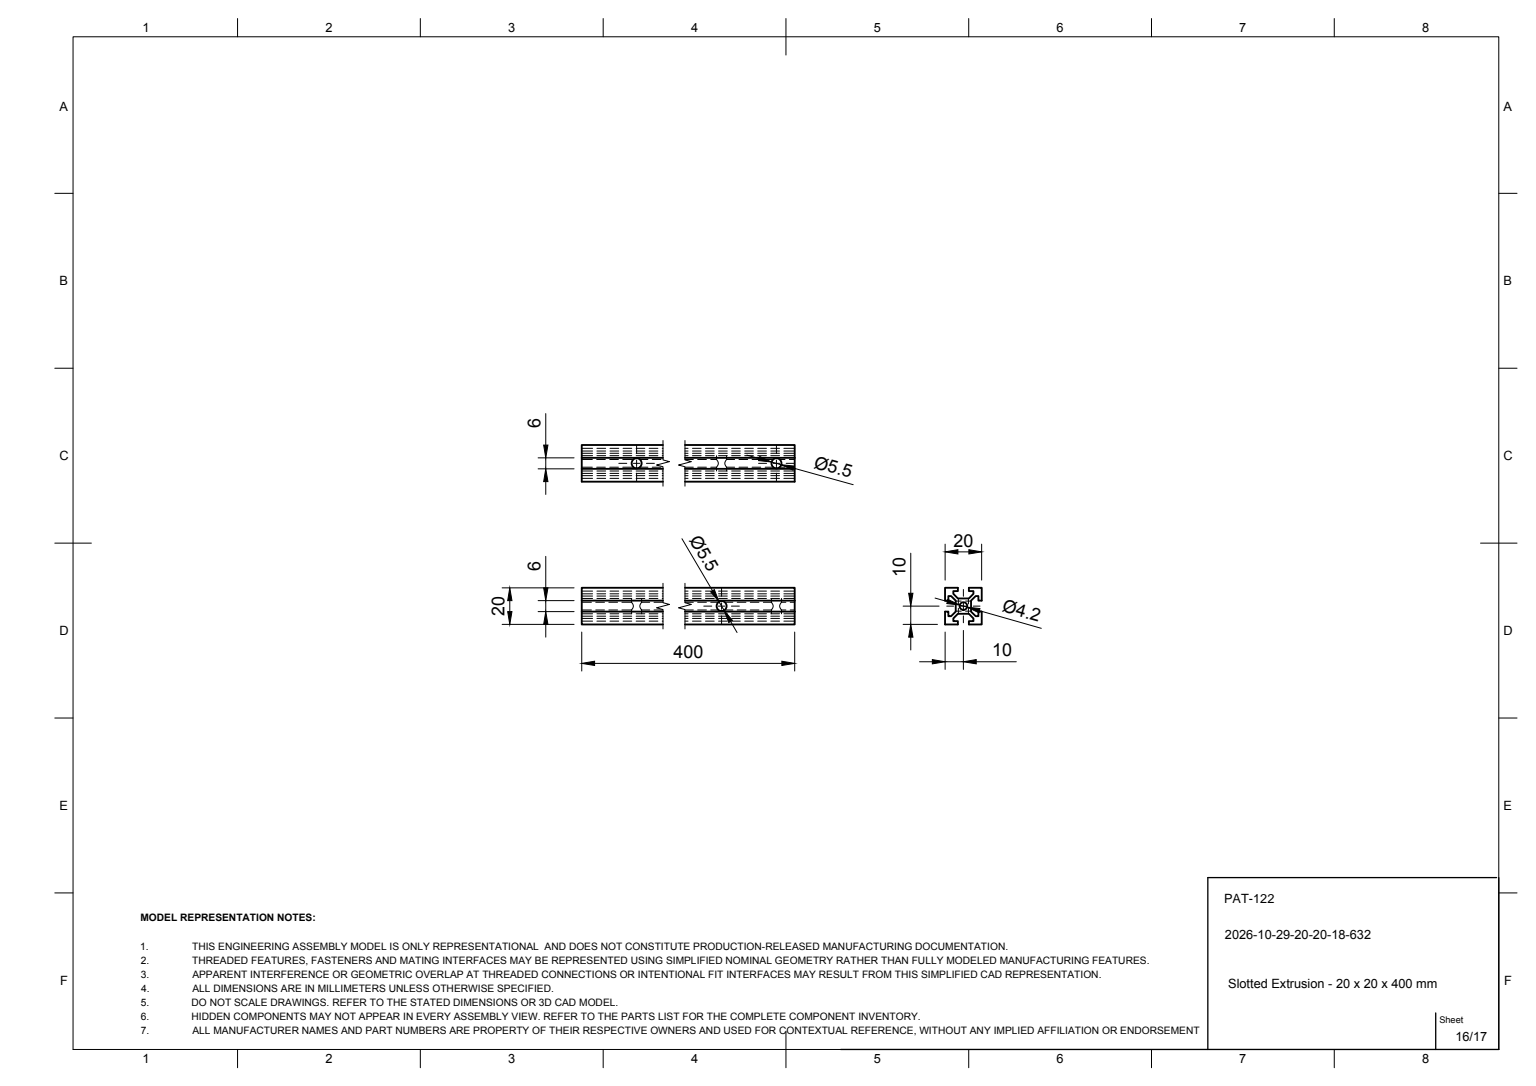
ISO-10303-21;
HEADER;
/* Generated by software containing ST-Developer
 * from STEP Tools, Inc. (www.steptools.com) 
 */

FILE_DESCRIPTION(
/* description */ ('PAT-122'),
/* implementation_level */ '2;1');

FILE_NAME(
/* name */ 'Slotted Extrusion - 20 x 20 x 400 mm.step',
/* time_stamp */ '2026-10-29T20:20:12-07:00',
/* author */ (''),
/* organization */ (''),
/* preprocessor_version */ 'ST-DEVELOPER v20.2',
/* originating_system */ 'Autodesk Translation Framework v15.17.0.0',
/* authorisation */ '');

FILE_SCHEMA (('AUTOMOTIVE_DESIGN { 1 0 10303 214 3 1 1 }'));
ENDSEC;

DATA;
#10=MECHANICAL_DESIGN_GEOMETRIC_PRESENTATION_REPRESENTATION('',(#504),#10019);
#425=B_SPLINE_CURVE_WITH_KNOTS('',3,(#8517,#8518,#8519,#8520,#8521,#8522,
#8523,#8524,#8525,#8526,#8527,#8528),.UNSPECIFIED.,.F.,.F.,(4,2,2,2,2,4),
(0.671876099962389,0.714365153473771,0.756854206985153,0.841832314007917,
0.92482323197575,1.00781414994358),.UNSPECIFIED.);
#426=B_SPLINE_CURVE_WITH_KNOTS('',3,(#8530,#8531,#8532,#8533,#8534,#8535,
#8536,#8537,#8538,#8539,#8540,#8541),.UNSPECIFIED.,.F.,.F.,(4,2,2,2,2,4),
(0.335938049981194,0.418928967949028,0.501919885916861,0.586897992939625,
0.629387046451007,0.671876099962389),.UNSPECIFIED.);
#427=B_SPLINE_CURVE_WITH_KNOTS('',3,(#8546,#8547,#8548,#8549,#8550,#8551,
#8552,#8553,#8554,#8555,#8556,#8557),.UNSPECIFIED.,.F.,.F.,(4,2,2,2,2,4),
(0.,0.042489053511382,0.0849781070227641,0.169956214045528,0.252947132013361,
0.335938049981194),.UNSPECIFIED.);
#428=B_SPLINE_CURVE_WITH_KNOTS('',3,(#8558,#8559,#8560,#8561,#8562,#8563,
#8564,#8565,#8566,#8567,#8568,#8569),.UNSPECIFIED.,.F.,.F.,(4,2,2,2,2,4),
(1.00781414994358,1.09080506791142,1.17379598587925,1.25877409290201,1.3012631464134,
1.34375219992478),.UNSPECIFIED.);
#429=B_SPLINE_CURVE_WITH_KNOTS('',3,(#8572,#8573,#8574,#8575,#8576,#8577,
#8578,#8579,#8580,#8581,#8582,#8583,#8584,#8585,#8586,#8587,#8588,#8589,
#8590,#8591,#8592,#8593),.UNSPECIFIED.,.F.,.F.,(4,2,2,2,2,2,2,2,2,2,4),
(0.,0.0424890535113821,0.0849781070227642,0.169956214045528,0.252947132013361,
0.335938049981194,0.418928967949028,0.501919885916861,0.586897992939625,
0.629387046451007,0.671876099962389),.UNSPECIFIED.);
#430=B_SPLINE_CURVE_WITH_KNOTS('',3,(#8594,#8595,#8596,#8597,#8598,#8599,
#8600,#8601,#8602,#8603,#8604,#8605,#8606,#8607,#8608,#8609,#8610,#8611,
#8612,#8613,#8614,#8615),.UNSPECIFIED.,.F.,.F.,(4,2,2,2,2,2,2,2,2,2,4),
(0.671876099962389,0.714365153473771,0.756854206985153,0.841832314007917,
0.92482323197575,1.00781414994358,1.09080506791142,1.17379598587925,1.25877409290201,
1.3012631464134,1.34375219992478),.UNSPECIFIED.);
#431=B_SPLINE_CURVE_WITH_KNOTS('',3,(#8622,#8623,#8624,#8625,#8626,#8627,
#8628,#8629,#8630,#8631,#8632,#8633),.UNSPECIFIED.,.F.,.F.,(4,2,2,2,2,4),
(0.67187609996239,0.714365153473772,0.756854206985154,0.841832314007918,
0.924823231975752,1.00781414994359),.UNSPECIFIED.);
#432=B_SPLINE_CURVE_WITH_KNOTS('',3,(#8635,#8636,#8637,#8638,#8639,#8640,
#8641,#8642,#8643,#8644,#8645,#8646),.UNSPECIFIED.,.F.,.F.,(4,2,2,2,2,4),
(0.335938049981195,0.418928967949029,0.501919885916863,0.586897992939627,
0.629387046451009,0.67187609996239),.UNSPECIFIED.);
#433=B_SPLINE_CURVE_WITH_KNOTS('',3,(#8651,#8652,#8653,#8654,#8655,#8656,
#8657,#8658,#8659,#8660,#8661,#8662),.UNSPECIFIED.,.F.,.F.,(4,2,2,2,2,4),
(0.,0.042489053511382,0.0849781070227639,0.169956214045528,0.252947132013362,
0.335938049981195),.UNSPECIFIED.);
#434=B_SPLINE_CURVE_WITH_KNOTS('',3,(#8663,#8664,#8665,#8666,#8667,#8668,
#8669,#8670,#8671,#8672,#8673,#8674),.UNSPECIFIED.,.F.,.F.,(4,2,2,2,2,4),
(1.00781414994359,1.09080506791142,1.17379598587925,1.25877409290202,1.3012631464134,
1.34375219992478),.UNSPECIFIED.);
#435=B_SPLINE_CURVE_WITH_KNOTS('',3,(#8677,#8678,#8679,#8680,#8681,#8682,
#8683,#8684,#8685,#8686,#8687,#8688,#8689,#8690,#8691,#8692,#8693,#8694,
#8695,#8696,#8697,#8698),.UNSPECIFIED.,.F.,.F.,(4,2,2,2,2,2,2,2,2,2,4),
(0.,0.042489053511382,0.084978107022764,0.169956214045528,0.252947132013362,
0.335938049981195,0.418928967949029,0.501919885916863,0.586897992939627,
0.629387046451009,0.671876099962391),.UNSPECIFIED.);
#436=B_SPLINE_CURVE_WITH_KNOTS('',3,(#8699,#8700,#8701,#8702,#8703,#8704,
#8705,#8706,#8707,#8708,#8709,#8710,#8711,#8712,#8713,#8714,#8715,#8716,
#8717,#8718,#8719,#8720),.UNSPECIFIED.,.F.,.F.,(4,2,2,2,2,2,2,2,2,2,4),
(0.671876099962391,0.714365153473772,0.756854206985154,0.841832314007918,
0.924823231975752,1.00781414994359,1.09080506791142,1.17379598587925,1.25877409290202,
1.3012631464134,1.34375219992478),.UNSPECIFIED.);
#437=B_SPLINE_CURVE_WITH_KNOTS('',3,(#8726,#8727,#8728,#8729,#8730,#8731,
#8732,#8733,#8734,#8735,#8736,#8737,#8738,#8739,#8740,#8741,#8742,#8743,
#8744,#8745,#8746,#8747,#8748,#8749,#8750,#8751,#8752,#8753,#8754,#8755,
#8756,#8757),.UNSPECIFIED.,.F.,.F.,(4,2,2,2,2,2,2,2,2,2,2,2,2,2,2,4),(0.,
0.0424890535113821,0.0849781070227642,0.169956214045528,0.252947132013362,
0.335938049981195,0.418928967949028,0.501919885916861,0.586897992939625,
0.629387046451007,0.67187609996239,0.714365153473772,0.756854206985154,
0.841832314007918,0.924823231975751,1.00781414994358),.UNSPECIFIED.);
#438=B_SPLINE_CURVE_WITH_KNOTS('',3,(#8759,#8760,#8761,#8762,#8763,#8764,
#8765,#8766,#8767,#8768,#8769,#8770),.UNSPECIFIED.,.F.,.F.,(4,2,2,2,2,4),
(1.00781414994358,1.09080506791142,1.17379598587925,1.25877409290201,1.3012631464134,
1.34375219992478),.UNSPECIFIED.);
#439=B_SPLINE_CURVE_WITH_KNOTS('',3,(#8777,#8778,#8779,#8780,#8781,#8782,
#8783,#8784,#8785,#8786,#8787,#8788,#8789,#8790,#8791,#8792,#8793,#8794,
#8795,#8796,#8797,#8798),.UNSPECIFIED.,.F.,.F.,(4,2,2,2,2,2,2,2,2,2,4),
(0.335938049981195,0.418928967949028,0.501919885916861,0.586897992939625,
0.629387046451007,0.671876099962389,0.714365153473771,0.756854206985153,
0.841832314007918,0.924823231975751,1.00781414994358),.UNSPECIFIED.);
#440=B_SPLINE_CURVE_WITH_KNOTS('',3,(#8803,#8804,#8805,#8806,#8807,#8808,
#8809,#8810,#8811,#8812,#8813,#8814),.UNSPECIFIED.,.F.,.F.,(4,2,2,2,2,4),
(0.,0.0424890535113821,0.0849781070227642,0.169956214045528,0.252947132013361,
0.335938049981195),.UNSPECIFIED.);
#441=B_SPLINE_CURVE_WITH_KNOTS('',3,(#8815,#8816,#8817,#8818,#8819,#8820,
#8821,#8822,#8823,#8824,#8825,#8826),.UNSPECIFIED.,.F.,.F.,(4,2,2,2,2,4),
(1.00781414994358,1.09080506791142,1.17379598587925,1.25877409290201,1.3012631464134,
1.34375219992478),.UNSPECIFIED.);
#442=B_SPLINE_CURVE_WITH_KNOTS('',3,(#8833,#8834,#8835,#8836,#8837,#8838,
#8839,#8840,#8841,#8842,#8843,#8844,#8845,#8846,#8847,#8848,#8849,#8850,
#8851,#8852,#8853,#8854),.UNSPECIFIED.,.F.,.F.,(4,2,2,2,2,2,2,2,2,2,4),
(0.335938049981195,0.418928967949029,0.501919885916863,0.586897992939627,
0.629387046451009,0.67187609996239,0.714365153473772,0.756854206985154,
0.841832314007918,0.924823231975752,1.00781414994359),.UNSPECIFIED.);
#443=B_SPLINE_CURVE_WITH_KNOTS('',3,(#8859,#8860,#8861,#8862,#8863,#8864,
#8865,#8866,#8867,#8868,#8869,#8870),.UNSPECIFIED.,.F.,.F.,(4,2,2,2,2,4),
(0.,0.042489053511382,0.0849781070227639,0.169956214045528,0.252947132013361,
0.335938049981195),.UNSPECIFIED.);
#444=B_SPLINE_CURVE_WITH_KNOTS('',3,(#8871,#8872,#8873,#8874,#8875,#8876,
#8877,#8878,#8879,#8880,#8881,#8882),.UNSPECIFIED.,.F.,.F.,(4,2,2,2,2,4),
(1.00781414994359,1.09080506791142,1.17379598587925,1.25877409290202,1.3012631464134,
1.34375219992478),.UNSPECIFIED.);
#445=B_SPLINE_CURVE_WITH_KNOTS('',3,(#8885,#8886,#8887,#8888,#8889,#8890,
#8891,#8892,#8893,#8894,#8895,#8896,#8897,#8898,#8899,#8900,#8901,#8902,
#8903,#8904,#8905,#8906,#8907,#8908,#8909,#8910,#8911,#8912,#8913,#8914,
#8915,#8916),.UNSPECIFIED.,.F.,.F.,(4,2,2,2,2,2,2,2,2,2,2,2,2,2,2,4),(0.,
0.042489053511382,0.084978107022764,0.169956214045528,0.252947132013362,
0.335938049981195,0.418928967949029,0.501919885916863,0.586897992939627,
0.629387046451009,0.671876099962391,0.714365153473772,0.756854206985154,
0.841832314007918,0.924823231975752,1.00781414994359),.UNSPECIFIED.);
#446=B_SPLINE_CURVE_WITH_KNOTS('',3,(#8917,#8918,#8919,#8920,#8921,#8922,
#8923,#8924,#8925,#8926,#8927,#8928),.UNSPECIFIED.,.F.,.F.,(4,2,2,2,2,4),
(1.00781414994359,1.09080506791142,1.17379598587925,1.25877409290202,1.3012631464134,
1.34375219992478),.UNSPECIFIED.);
#460=SHAPE_REPRESENTATION_RELATIONSHIP('SRR','None',#10181,#482);
#482=ADVANCED_BREP_SHAPE_REPRESENTATION('',(#526),#10010);
#504=STYLED_ITEM('',(#10334),#526);
#526=MANIFOLD_SOLID_BREP('Body1',#5626);
#583=FACE_BOUND('',#1268,.T.);
#584=FACE_BOUND('',#1270,.T.);
#585=FACE_BOUND('',#1274,.T.);
#586=FACE_BOUND('',#1276,.T.);
#587=FACE_BOUND('',#1284,.T.);
#588=FACE_BOUND('',#1285,.T.);
#589=FACE_BOUND('',#1295,.T.);
#590=FACE_BOUND('',#1296,.T.);
#591=FACE_BOUND('',#1306,.T.);
#592=FACE_BOUND('',#1307,.T.);
#593=FACE_BOUND('',#1317,.T.);
#594=FACE_BOUND('',#1318,.T.);
#595=FACE_BOUND('',#1333,.T.);
#596=FACE_BOUND('',#1335,.T.);
#671=PLANE('',#6084);
#672=PLANE('',#6085);
#673=PLANE('',#6086);
#674=PLANE('',#6087);
#675=PLANE('',#6088);
#676=PLANE('',#6089);
#677=PLANE('',#6090);
#678=PLANE('',#6091);
#679=PLANE('',#6092);
#680=PLANE('',#6093);
#681=PLANE('',#6094);
#682=PLANE('',#6095);
#683=PLANE('',#6096);
#684=PLANE('',#6097);
#685=PLANE('',#6098);
#686=PLANE('',#6099);
#687=PLANE('',#6100);
#688=PLANE('',#6101);
#689=PLANE('',#6102);
#690=PLANE('',#6103);
#691=PLANE('',#6104);
#692=PLANE('',#6105);
#693=PLANE('',#6106);
#694=PLANE('',#6107);
#695=PLANE('',#6108);
#696=PLANE('',#6109);
#697=PLANE('',#6110);
#698=PLANE('',#6111);
#699=PLANE('',#6112);
#700=PLANE('',#6113);
#701=PLANE('',#6114);
#702=PLANE('',#6115);
#703=PLANE('',#6116);
#704=PLANE('',#6117);
#705=PLANE('',#6118);
#706=PLANE('',#6119);
#707=PLANE('',#6122);
#708=PLANE('',#6123);
#709=PLANE('',#6124);
#710=PLANE('',#6125);
#711=PLANE('',#6126);
#712=PLANE('',#6127);
#713=PLANE('',#6128);
#714=PLANE('',#6129);
#715=PLANE('',#6130);
#716=PLANE('',#6131);
#923=FACE_OUTER_BOUND('',#1267,.T.);
#924=FACE_OUTER_BOUND('',#1269,.T.);
#925=FACE_OUTER_BOUND('',#1271,.T.);
#926=FACE_OUTER_BOUND('',#1272,.T.);
#927=FACE_OUTER_BOUND('',#1273,.T.);
#928=FACE_OUTER_BOUND('',#1275,.T.);
#929=FACE_OUTER_BOUND('',#1277,.T.);
#930=FACE_OUTER_BOUND('',#1278,.T.);
#931=FACE_OUTER_BOUND('',#1279,.T.);
#932=FACE_OUTER_BOUND('',#1280,.T.);
#933=FACE_OUTER_BOUND('',#1281,.T.);
#934=FACE_OUTER_BOUND('',#1282,.T.);
#935=FACE_OUTER_BOUND('',#1283,.T.);
#936=FACE_OUTER_BOUND('',#1286,.T.);
#937=FACE_OUTER_BOUND('',#1287,.T.);
#938=FACE_OUTER_BOUND('',#1288,.T.);
#939=FACE_OUTER_BOUND('',#1289,.T.);
#940=FACE_OUTER_BOUND('',#1290,.T.);
#941=FACE_OUTER_BOUND('',#1291,.T.);
#942=FACE_OUTER_BOUND('',#1292,.T.);
#943=FACE_OUTER_BOUND('',#1293,.T.);
#944=FACE_OUTER_BOUND('',#1294,.T.);
#945=FACE_OUTER_BOUND('',#1297,.T.);
#946=FACE_OUTER_BOUND('',#1298,.T.);
#947=FACE_OUTER_BOUND('',#1299,.T.);
#948=FACE_OUTER_BOUND('',#1300,.T.);
#949=FACE_OUTER_BOUND('',#1301,.T.);
#950=FACE_OUTER_BOUND('',#1302,.T.);
#951=FACE_OUTER_BOUND('',#1303,.T.);
#952=FACE_OUTER_BOUND('',#1304,.T.);
#953=FACE_OUTER_BOUND('',#1305,.T.);
#954=FACE_OUTER_BOUND('',#1308,.T.);
#955=FACE_OUTER_BOUND('',#1309,.T.);
#956=FACE_OUTER_BOUND('',#1310,.T.);
#957=FACE_OUTER_BOUND('',#1311,.T.);
#958=FACE_OUTER_BOUND('',#1312,.T.);
#959=FACE_OUTER_BOUND('',#1313,.T.);
#960=FACE_OUTER_BOUND('',#1314,.T.);
#961=FACE_OUTER_BOUND('',#1315,.T.);
#962=FACE_OUTER_BOUND('',#1316,.T.);
#963=FACE_OUTER_BOUND('',#1319,.T.);
#964=FACE_OUTER_BOUND('',#1320,.T.);
#965=FACE_OUTER_BOUND('',#1321,.T.);
#966=FACE_OUTER_BOUND('',#1322,.T.);
#967=FACE_OUTER_BOUND('',#1323,.T.);
#968=FACE_OUTER_BOUND('',#1324,.T.);
#969=FACE_OUTER_BOUND('',#1325,.T.);
#970=FACE_OUTER_BOUND('',#1326,.T.);
#971=FACE_OUTER_BOUND('',#1327,.T.);
#972=FACE_OUTER_BOUND('',#1328,.T.);
#973=FACE_OUTER_BOUND('',#1329,.T.);
#974=FACE_OUTER_BOUND('',#1330,.T.);
#975=FACE_OUTER_BOUND('',#1331,.T.);
#976=FACE_OUTER_BOUND('',#1332,.T.);
#977=FACE_OUTER_BOUND('',#1334,.T.);
#1267=EDGE_LOOP('',(#4273,#4274,#4275,#4276,#4277,#4278,#4279,#4280,#4281,
#4282));
#1268=EDGE_LOOP('',(#4283,#4284));
#1269=EDGE_LOOP('',(#4285,#4286,#4287,#4288,#4289,#4290,#4291,#4292,#4293,
#4294));
#1270=EDGE_LOOP('',(#4295,#4296));
#1271=EDGE_LOOP('',(#4297,#4298,#4299,#4300,#4301,#4302,#4303,#4304));
#1272=EDGE_LOOP('',(#4305,#4306,#4307,#4308,#4309,#4310,#4311,#4312));
#1273=EDGE_LOOP('',(#4313,#4314,#4315,#4316,#4317,#4318,#4319,#4320,#4321));
#1274=EDGE_LOOP('',(#4322,#4323));
#1275=EDGE_LOOP('',(#4324,#4325,#4326,#4327,#4328,#4329,#4330,#4331,#4332));
#1276=EDGE_LOOP('',(#4333,#4334));
#1277=EDGE_LOOP('',(#4335,#4336,#4337,#4338,#4339,#4340,#4341));
#1278=EDGE_LOOP('',(#4342,#4343,#4344,#4345,#4346,#4347));
#1279=EDGE_LOOP('',(#4348,#4349,#4350,#4351));
#1280=EDGE_LOOP('',(#4352,#4353,#4354,#4355));
#1281=EDGE_LOOP('',(#4356,#4357,#4358,#4359));
#1282=EDGE_LOOP('',(#4360,#4361,#4362,#4363));
#1283=EDGE_LOOP('',(#4364,#4365,#4366,#4367));
#1284=EDGE_LOOP('',(#4368));
#1285=EDGE_LOOP('',(#4369));
#1286=EDGE_LOOP('',(#4370,#4371,#4372,#4373));
#1287=EDGE_LOOP('',(#4374,#4375,#4376,#4377));
#1288=EDGE_LOOP('',(#4378,#4379,#4380,#4381));
#1289=EDGE_LOOP('',(#4382,#4383,#4384,#4385));
#1290=EDGE_LOOP('',(#4386,#4387,#4388,#4389));
#1291=EDGE_LOOP('',(#4390,#4391,#4392,#4393));
#1292=EDGE_LOOP('',(#4394,#4395,#4396,#4397));
#1293=EDGE_LOOP('',(#4398,#4399,#4400,#4401));
#1294=EDGE_LOOP('',(#4402,#4403,#4404,#4405));
#1295=EDGE_LOOP('',(#4406));
#1296=EDGE_LOOP('',(#4407));
#1297=EDGE_LOOP('',(#4408,#4409,#4410,#4411));
#1298=EDGE_LOOP('',(#4412,#4413,#4414,#4415));
#1299=EDGE_LOOP('',(#4416,#4417,#4418,#4419));
#1300=EDGE_LOOP('',(#4420,#4421,#4422,#4423));
#1301=EDGE_LOOP('',(#4424,#4425,#4426,#4427));
#1302=EDGE_LOOP('',(#4428,#4429,#4430,#4431));
#1303=EDGE_LOOP('',(#4432,#4433,#4434,#4435));
#1304=EDGE_LOOP('',(#4436,#4437,#4438,#4439));
#1305=EDGE_LOOP('',(#4440,#4441,#4442,#4443));
#1306=EDGE_LOOP('',(#4444));
#1307=EDGE_LOOP('',(#4445));
#1308=EDGE_LOOP('',(#4446,#4447,#4448,#4449));
#1309=EDGE_LOOP('',(#4450,#4451,#4452,#4453));
#1310=EDGE_LOOP('',(#4454,#4455,#4456,#4457));
#1311=EDGE_LOOP('',(#4458,#4459,#4460,#4461));
#1312=EDGE_LOOP('',(#4462,#4463,#4464,#4465));
#1313=EDGE_LOOP('',(#4466,#4467,#4468,#4469));
#1314=EDGE_LOOP('',(#4470,#4471,#4472,#4473));
#1315=EDGE_LOOP('',(#4474,#4475,#4476,#4477));
#1316=EDGE_LOOP('',(#4478,#4479,#4480,#4481));
#1317=EDGE_LOOP('',(#4482));
#1318=EDGE_LOOP('',(#4483));
#1319=EDGE_LOOP('',(#4484,#4485,#4486,#4487));
#1320=EDGE_LOOP('',(#4488,#4489,#4490,#4491));
#1321=EDGE_LOOP('',(#4492,#4493,#4494,#4495));
#1322=EDGE_LOOP('',(#4496,#4497,#4498,#4499));
#1323=EDGE_LOOP('',(#4500,#4501,#4502,#4503,#4504));
#1324=EDGE_LOOP('',(#4505,#4506,#4507,#4508));
#1325=EDGE_LOOP('',(#4509,#4510,#4511,#4512));
#1326=EDGE_LOOP('',(#4513,#4514,#4515,#4516));
#1327=EDGE_LOOP('',(#4517,#4518,#4519,#4520));
#1328=EDGE_LOOP('',(#4521,#4522,#4523,#4524));
#1329=EDGE_LOOP('',(#4525,#4526,#4527,#4528));
#1330=EDGE_LOOP('',(#4529,#4530,#4531,#4532));
#1331=EDGE_LOOP('',(#4533,#4534,#4535,#4536));
#1332=EDGE_LOOP('',(#4537,#4538,#4539,#4540,#4541,#4542,#4543,#4544,#4545,
#4546,#4547,#4548,#4549,#4550,#4551,#4552,#4553,#4554,#4555,#4556,#4557,
#4558,#4559,#4560,#4561,#4562,#4563,#4564,#4565,#4566,#4567,#4568,#4569,
#4570,#4571,#4572,#4573,#4574,#4575,#4576,#4577,#4578,#4579,#4580));
#1333=EDGE_LOOP('',(#4581));
#1334=EDGE_LOOP('',(#4582,#4583,#4584,#4585,#4586,#4587,#4588,#4589,#4590,
#4591,#4592,#4593,#4594,#4595,#4596,#4597,#4598,#4599,#4600,#4601,#4602,
#4603,#4604,#4605,#4606,#4607,#4608,#4609,#4610,#4611,#4612,#4613,#4614,
#4615,#4616,#4617,#4618,#4619,#4620,#4621,#4622,#4623,#4624,#4625));
#1335=EDGE_LOOP('',(#4626));
#1619=LINE('',#8515,#2163);
#1620=LINE('',#8543,#2164);
#1621=LINE('',#8620,#2165);
#1622=LINE('',#8648,#2166);
#1623=LINE('',#8722,#2167);
#1624=LINE('',#8758,#2168);
#1625=LINE('',#8775,#2169);
#1626=LINE('',#8800,#2170);
#1627=LINE('',#8831,#2171);
#1628=LINE('',#8856,#2172);
#1629=LINE('',#8930,#2173);
#1630=LINE('',#8934,#2174);
#1631=LINE('',#8938,#2175);
#1632=LINE('',#8940,#2176);
#1633=LINE('',#8942,#2177);
#1634=LINE('',#8943,#2178);
#1635=LINE('',#8946,#2179);
#1636=LINE('',#8948,#2180);
#1637=LINE('',#8949,#2181);
#1638=LINE('',#8952,#2182);
#1639=LINE('',#8954,#2183);
#1640=LINE('',#8955,#2184);
#1641=LINE('',#8958,#2185);
#1642=LINE('',#8960,#2186);
#1643=LINE('',#8961,#2187);
#1644=LINE('',#8964,#2188);
#1645=LINE('',#8966,#2189);
#1646=LINE('',#8967,#2190);
#1647=LINE('',#8970,#2191);
#1648=LINE('',#8972,#2192);
#1649=LINE('',#8973,#2193);
#1650=LINE('',#8976,#2194);
#1651=LINE('',#8978,#2195);
#1652=LINE('',#8979,#2196);
#1653=LINE('',#8982,#2197);
#1654=LINE('',#8984,#2198);
#1655=LINE('',#8985,#2199);
#1656=LINE('',#8988,#2200);
#1657=LINE('',#8990,#2201);
#1658=LINE('',#8991,#2202);
#1659=LINE('',#8995,#2203);
#1660=LINE('',#8997,#2204);
#1661=LINE('',#8999,#2205);
#1662=LINE('',#9000,#2206);
#1663=LINE('',#9003,#2207);
#1664=LINE('',#9005,#2208);
#1665=LINE('',#9006,#2209);
#1666=LINE('',#9009,#2210);
#1667=LINE('',#9011,#2211);
#1668=LINE('',#9012,#2212);
#1669=LINE('',#9015,#2213);
#1670=LINE('',#9017,#2214);
#1671=LINE('',#9018,#2215);
#1672=LINE('',#9021,#2216);
#1673=LINE('',#9023,#2217);
#1674=LINE('',#9024,#2218);
#1675=LINE('',#9027,#2219);
#1676=LINE('',#9029,#2220);
#1677=LINE('',#9030,#2221);
#1678=LINE('',#9033,#2222);
#1679=LINE('',#9035,#2223);
#1680=LINE('',#9036,#2224);
#1681=LINE('',#9039,#2225);
#1682=LINE('',#9041,#2226);
#1683=LINE('',#9042,#2227);
#1684=LINE('',#9045,#2228);
#1685=LINE('',#9047,#2229);
#1686=LINE('',#9048,#2230);
#1687=LINE('',#9052,#2231);
#1688=LINE('',#9054,#2232);
#1689=LINE('',#9056,#2233);
#1690=LINE('',#9057,#2234);
#1691=LINE('',#9060,#2235);
#1692=LINE('',#9062,#2236);
#1693=LINE('',#9063,#2237);
#1694=LINE('',#9066,#2238);
#1695=LINE('',#9068,#2239);
#1696=LINE('',#9069,#2240);
#1697=LINE('',#9072,#2241);
#1698=LINE('',#9074,#2242);
#1699=LINE('',#9075,#2243);
#1700=LINE('',#9078,#2244);
#1701=LINE('',#9080,#2245);
#1702=LINE('',#9081,#2246);
#1703=LINE('',#9084,#2247);
#1704=LINE('',#9086,#2248);
#1705=LINE('',#9087,#2249);
#1706=LINE('',#9090,#2250);
#1707=LINE('',#9092,#2251);
#1708=LINE('',#9093,#2252);
#1709=LINE('',#9096,#2253);
#1710=LINE('',#9098,#2254);
#1711=LINE('',#9099,#2255);
#1712=LINE('',#9102,#2256);
#1713=LINE('',#9104,#2257);
#1714=LINE('',#9105,#2258);
#1715=LINE('',#9109,#2259);
#1716=LINE('',#9111,#2260);
#1717=LINE('',#9113,#2261);
#1718=LINE('',#9114,#2262);
#1719=LINE('',#9117,#2263);
#1720=LINE('',#9119,#2264);
#1721=LINE('',#9120,#2265);
#1722=LINE('',#9123,#2266);
#1723=LINE('',#9125,#2267);
#1724=LINE('',#9126,#2268);
#1725=LINE('',#9129,#2269);
#1726=LINE('',#9131,#2270);
#1727=LINE('',#9132,#2271);
#1728=LINE('',#9135,#2272);
#1729=LINE('',#9137,#2273);
#1730=LINE('',#9138,#2274);
#1731=LINE('',#9141,#2275);
#1732=LINE('',#9143,#2276);
#1733=LINE('',#9144,#2277);
#1734=LINE('',#9147,#2278);
#1735=LINE('',#9149,#2279);
#1736=LINE('',#9150,#2280);
#1737=LINE('',#9153,#2281);
#1738=LINE('',#9155,#2282);
#1739=LINE('',#9156,#2283);
#1740=LINE('',#9159,#2284);
#1741=LINE('',#9161,#2285);
#1742=LINE('',#9162,#2286);
#1743=LINE('',#9165,#2287);
#1744=LINE('',#9169,#2288);
#1745=LINE('',#9171,#2289);
#1746=LINE('',#9172,#2290);
#1747=LINE('',#9175,#2291);
#1748=LINE('',#9177,#2292);
#1749=LINE('',#9178,#2293);
#1750=LINE('',#9180,#2294);
#1751=LINE('',#9181,#2295);
#1752=LINE('',#9184,#2296);
#1753=LINE('',#9186,#2297);
#1754=LINE('',#9187,#2298);
#1755=LINE('',#9189,#2299);
#1756=LINE('',#9190,#2300);
#1757=LINE('',#9193,#2301);
#1758=LINE('',#9195,#2302);
#1759=LINE('',#9196,#2303);
#1760=LINE('',#9198,#2304);
#1761=LINE('',#9199,#2305);
#1762=LINE('',#9201,#2306);
#1763=LINE('',#9202,#2307);
#2163=VECTOR('',#6932,0.275);
#2164=VECTOR('',#6933,0.275);
#2165=VECTOR('',#6940,0.274999999999999);
#2166=VECTOR('',#6941,0.274999999999999);
#2167=VECTOR('',#6946,0.21);
#2168=VECTOR('',#6949,0.21);
#2169=VECTOR('',#6954,0.275);
#2170=VECTOR('',#6955,0.275);
#2171=VECTOR('',#6962,0.274999999999999);
#2172=VECTOR('',#6963,0.274999999999999);
#2173=VECTOR('',#6968,0.21);
#2174=VECTOR('',#6973,0.21);
#2175=VECTOR('',#6976,1.);
#2176=VECTOR('',#6977,1.);
#2177=VECTOR('',#6978,1.);
#2178=VECTOR('',#6979,1.);
#2179=VECTOR('',#6982,1.);
#2180=VECTOR('',#6983,1.);
#2181=VECTOR('',#6984,1.);
#2182=VECTOR('',#6987,1.);
#2183=VECTOR('',#6988,1.);
#2184=VECTOR('',#6989,1.);
#2185=VECTOR('',#6992,1.);
#2186=VECTOR('',#6993,1.);
#2187=VECTOR('',#6994,1.);
#2188=VECTOR('',#6997,1.);
#2189=VECTOR('',#6998,1.);
#2190=VECTOR('',#6999,1.);
#2191=VECTOR('',#7002,1.);
#2192=VECTOR('',#7003,1.);
#2193=VECTOR('',#7004,1.);
#2194=VECTOR('',#7007,1.);
#2195=VECTOR('',#7008,1.);
#2196=VECTOR('',#7009,1.);
#2197=VECTOR('',#7012,1.);
#2198=VECTOR('',#7013,1.);
#2199=VECTOR('',#7014,1.);
#2200=VECTOR('',#7017,1.);
#2201=VECTOR('',#7018,1.);
#2202=VECTOR('',#7019,1.);
#2203=VECTOR('',#7022,1.);
#2204=VECTOR('',#7023,1.);
#2205=VECTOR('',#7024,1.);
#2206=VECTOR('',#7025,1.);
#2207=VECTOR('',#7028,1.);
#2208=VECTOR('',#7029,1.);
#2209=VECTOR('',#7030,1.);
#2210=VECTOR('',#7033,1.);
#2211=VECTOR('',#7034,1.);
#2212=VECTOR('',#7035,1.);
#2213=VECTOR('',#7038,1.);
#2214=VECTOR('',#7039,1.);
#2215=VECTOR('',#7040,1.);
#2216=VECTOR('',#7043,1.);
#2217=VECTOR('',#7044,1.);
#2218=VECTOR('',#7045,1.);
#2219=VECTOR('',#7048,1.);
#2220=VECTOR('',#7049,1.);
#2221=VECTOR('',#7050,1.);
#2222=VECTOR('',#7053,1.);
#2223=VECTOR('',#7054,1.);
#2224=VECTOR('',#7055,1.);
#2225=VECTOR('',#7058,1.);
#2226=VECTOR('',#7059,1.);
#2227=VECTOR('',#7060,1.);
#2228=VECTOR('',#7063,1.);
#2229=VECTOR('',#7064,1.);
#2230=VECTOR('',#7065,1.);
#2231=VECTOR('',#7068,1.);
#2232=VECTOR('',#7069,1.);
#2233=VECTOR('',#7070,1.);
#2234=VECTOR('',#7071,1.);
#2235=VECTOR('',#7074,1.);
#2236=VECTOR('',#7075,1.);
#2237=VECTOR('',#7076,1.);
#2238=VECTOR('',#7079,1.);
#2239=VECTOR('',#7080,1.);
#2240=VECTOR('',#7081,1.);
#2241=VECTOR('',#7084,1.);
#2242=VECTOR('',#7085,1.);
#2243=VECTOR('',#7086,1.);
#2244=VECTOR('',#7089,1.);
#2245=VECTOR('',#7090,1.);
#2246=VECTOR('',#7091,1.);
#2247=VECTOR('',#7094,1.);
#2248=VECTOR('',#7095,1.);
#2249=VECTOR('',#7096,1.);
#2250=VECTOR('',#7099,1.);
#2251=VECTOR('',#7100,1.);
#2252=VECTOR('',#7101,1.);
#2253=VECTOR('',#7104,1.);
#2254=VECTOR('',#7105,1.);
#2255=VECTOR('',#7106,1.);
#2256=VECTOR('',#7109,1.);
#2257=VECTOR('',#7110,1.);
#2258=VECTOR('',#7111,1.);
#2259=VECTOR('',#7114,1.);
#2260=VECTOR('',#7115,1.);
#2261=VECTOR('',#7116,1.);
#2262=VECTOR('',#7117,1.);
#2263=VECTOR('',#7120,1.);
#2264=VECTOR('',#7121,1.);
#2265=VECTOR('',#7122,1.);
#2266=VECTOR('',#7125,1.);
#2267=VECTOR('',#7126,1.);
#2268=VECTOR('',#7127,1.);
#2269=VECTOR('',#7130,1.);
#2270=VECTOR('',#7131,1.);
#2271=VECTOR('',#7132,1.);
#2272=VECTOR('',#7135,1.);
#2273=VECTOR('',#7136,1.);
#2274=VECTOR('',#7137,1.);
#2275=VECTOR('',#7140,1.);
#2276=VECTOR('',#7141,1.);
#2277=VECTOR('',#7142,1.);
#2278=VECTOR('',#7145,1.);
#2279=VECTOR('',#7146,1.);
#2280=VECTOR('',#7147,1.);
#2281=VECTOR('',#7150,1.);
#2282=VECTOR('',#7151,1.);
#2283=VECTOR('',#7152,1.);
#2284=VECTOR('',#7155,1.);
#2285=VECTOR('',#7156,1.);
#2286=VECTOR('',#7157,1.);
#2287=VECTOR('',#7160,0.21);
#2288=VECTOR('',#7165,1.);
#2289=VECTOR('',#7166,1.);
#2290=VECTOR('',#7167,1.);
#2291=VECTOR('',#7170,1.);
#2292=VECTOR('',#7171,1.);
#2293=VECTOR('',#7172,1.);
#2294=VECTOR('',#7175,1.);
#2295=VECTOR('',#7176,1.);
#2296=VECTOR('',#7179,1.);
#2297=VECTOR('',#7180,1.);
#2298=VECTOR('',#7181,1.);
#2299=VECTOR('',#7184,1.);
#2300=VECTOR('',#7185,1.);
#2301=VECTOR('',#7188,1.);
#2302=VECTOR('',#7189,1.);
#2303=VECTOR('',#7190,1.);
#2304=VECTOR('',#7193,1.);
#2305=VECTOR('',#7194,1.);
#2306=VECTOR('',#7197,1.);
#2307=VECTOR('',#7198,1.);
#2647=CIRCLE('',#6068,0.275);
#2648=CIRCLE('',#6069,0.275);
#2649=CIRCLE('',#6071,0.274999999999999);
#2650=CIRCLE('',#6072,0.274999999999999);
#2651=CIRCLE('',#6076,0.275);
#2652=CIRCLE('',#6077,0.275);
#2653=CIRCLE('',#6079,0.274999999999999);
#2654=CIRCLE('',#6080,0.274999999999999);
#2655=CIRCLE('',#6083,0.21);
#2656=CIRCLE('',#6121,0.21);
#2841=VERTEX_POINT('',#8512);
#2842=VERTEX_POINT('',#8514);
#2843=VERTEX_POINT('',#8516);
#2844=VERTEX_POINT('',#8529);
#2845=VERTEX_POINT('',#8542);
#2846=VERTEX_POINT('',#8545);
#2847=VERTEX_POINT('',#8570);
#2848=VERTEX_POINT('',#8571);
#2849=VERTEX_POINT('',#8617);
#2850=VERTEX_POINT('',#8619);
#2851=VERTEX_POINT('',#8621);
#2852=VERTEX_POINT('',#8634);
#2853=VERTEX_POINT('',#8647);
#2854=VERTEX_POINT('',#8650);
#2855=VERTEX_POINT('',#8675);
#2856=VERTEX_POINT('',#8676);
#2857=VERTEX_POINT('',#8724);
#2858=VERTEX_POINT('',#8725);
#2859=VERTEX_POINT('',#8772);
#2860=VERTEX_POINT('',#8774);
#2861=VERTEX_POINT('',#8776);
#2862=VERTEX_POINT('',#8799);
#2863=VERTEX_POINT('',#8802);
#2864=VERTEX_POINT('',#8828);
#2865=VERTEX_POINT('',#8830);
#2866=VERTEX_POINT('',#8832);
#2867=VERTEX_POINT('',#8855);
#2868=VERTEX_POINT('',#8858);
#2869=VERTEX_POINT('',#8883);
#2870=VERTEX_POINT('',#8884);
#2871=VERTEX_POINT('',#8932);
#2872=VERTEX_POINT('',#8936);
#2873=VERTEX_POINT('',#8937);
#2874=VERTEX_POINT('',#8939);
#2875=VERTEX_POINT('',#8941);
#2876=VERTEX_POINT('',#8945);
#2877=VERTEX_POINT('',#8947);
#2878=VERTEX_POINT('',#8951);
#2879=VERTEX_POINT('',#8953);
#2880=VERTEX_POINT('',#8957);
#2881=VERTEX_POINT('',#8959);
#2882=VERTEX_POINT('',#8963);
#2883=VERTEX_POINT('',#8965);
#2884=VERTEX_POINT('',#8969);
#2885=VERTEX_POINT('',#8971);
#2886=VERTEX_POINT('',#8975);
#2887=VERTEX_POINT('',#8977);
#2888=VERTEX_POINT('',#8981);
#2889=VERTEX_POINT('',#8983);
#2890=VERTEX_POINT('',#8987);
#2891=VERTEX_POINT('',#8989);
#2892=VERTEX_POINT('',#8993);
#2893=VERTEX_POINT('',#8994);
#2894=VERTEX_POINT('',#8996);
#2895=VERTEX_POINT('',#8998);
#2896=VERTEX_POINT('',#9002);
#2897=VERTEX_POINT('',#9004);
#2898=VERTEX_POINT('',#9008);
#2899=VERTEX_POINT('',#9010);
#2900=VERTEX_POINT('',#9014);
#2901=VERTEX_POINT('',#9016);
#2902=VERTEX_POINT('',#9020);
#2903=VERTEX_POINT('',#9022);
#2904=VERTEX_POINT('',#9026);
#2905=VERTEX_POINT('',#9028);
#2906=VERTEX_POINT('',#9032);
#2907=VERTEX_POINT('',#9034);
#2908=VERTEX_POINT('',#9038);
#2909=VERTEX_POINT('',#9040);
#2910=VERTEX_POINT('',#9044);
#2911=VERTEX_POINT('',#9046);
#2912=VERTEX_POINT('',#9050);
#2913=VERTEX_POINT('',#9051);
#2914=VERTEX_POINT('',#9053);
#2915=VERTEX_POINT('',#9055);
#2916=VERTEX_POINT('',#9059);
#2917=VERTEX_POINT('',#9061);
#2918=VERTEX_POINT('',#9065);
#2919=VERTEX_POINT('',#9067);
#2920=VERTEX_POINT('',#9071);
#2921=VERTEX_POINT('',#9073);
#2922=VERTEX_POINT('',#9077);
#2923=VERTEX_POINT('',#9079);
#2924=VERTEX_POINT('',#9083);
#2925=VERTEX_POINT('',#9085);
#2926=VERTEX_POINT('',#9089);
#2927=VERTEX_POINT('',#9091);
#2928=VERTEX_POINT('',#9095);
#2929=VERTEX_POINT('',#9097);
#2930=VERTEX_POINT('',#9101);
#2931=VERTEX_POINT('',#9103);
#2932=VERTEX_POINT('',#9107);
#2933=VERTEX_POINT('',#9108);
#2934=VERTEX_POINT('',#9110);
#2935=VERTEX_POINT('',#9112);
#2936=VERTEX_POINT('',#9116);
#2937=VERTEX_POINT('',#9118);
#2938=VERTEX_POINT('',#9122);
#2939=VERTEX_POINT('',#9124);
#2940=VERTEX_POINT('',#9128);
#2941=VERTEX_POINT('',#9130);
#2942=VERTEX_POINT('',#9134);
#2943=VERTEX_POINT('',#9136);
#2944=VERTEX_POINT('',#9140);
#2945=VERTEX_POINT('',#9142);
#2946=VERTEX_POINT('',#9146);
#2947=VERTEX_POINT('',#9148);
#2948=VERTEX_POINT('',#9152);
#2949=VERTEX_POINT('',#9154);
#2950=VERTEX_POINT('',#9158);
#2951=VERTEX_POINT('',#9160);
#2952=VERTEX_POINT('',#9164);
#2953=VERTEX_POINT('',#9168);
#2954=VERTEX_POINT('',#9170);
#2955=VERTEX_POINT('',#9174);
#2956=VERTEX_POINT('',#9176);
#2957=VERTEX_POINT('',#9183);
#2958=VERTEX_POINT('',#9185);
#2959=VERTEX_POINT('',#9192);
#2960=VERTEX_POINT('',#9194);
#3371=EDGE_CURVE('',#2841,#2841,#2647,.T.);
#3372=EDGE_CURVE('',#2841,#2842,#1619,.T.);
#3373=EDGE_CURVE('',#2843,#2842,#425,.T.);
#3374=EDGE_CURVE('',#2844,#2843,#426,.T.);
#3375=EDGE_CURVE('',#2844,#2845,#1620,.T.);
#3376=EDGE_CURVE('',#2845,#2845,#2648,.T.);
#3377=EDGE_CURVE('',#2846,#2844,#427,.T.);
#3378=EDGE_CURVE('',#2842,#2846,#428,.T.);
#3379=EDGE_CURVE('',#2847,#2848,#429,.T.);
#3380=EDGE_CURVE('',#2848,#2847,#430,.T.);
#3381=EDGE_CURVE('',#2849,#2849,#2649,.T.);
#3382=EDGE_CURVE('',#2849,#2850,#1621,.T.);
#3383=EDGE_CURVE('',#2851,#2850,#431,.T.);
#3384=EDGE_CURVE('',#2852,#2851,#432,.T.);
#3385=EDGE_CURVE('',#2852,#2853,#1622,.T.);
#3386=EDGE_CURVE('',#2853,#2853,#2650,.T.);
#3387=EDGE_CURVE('',#2854,#2852,#433,.T.);
#3388=EDGE_CURVE('',#2850,#2854,#434,.T.);
#3389=EDGE_CURVE('',#2855,#2856,#435,.T.);
#3390=EDGE_CURVE('',#2856,#2855,#436,.T.);
#3391=EDGE_CURVE('',#2848,#2851,#1623,.T.);
#3392=EDGE_CURVE('',#2857,#2858,#437,.T.);
#3393=EDGE_CURVE('',#2858,#2843,#1624,.T.);
#3394=EDGE_CURVE('',#2858,#2857,#438,.T.);
#3395=EDGE_CURVE('',#2859,#2859,#2651,.T.);
#3396=EDGE_CURVE('',#2859,#2860,#1625,.T.);
#3397=EDGE_CURVE('',#2861,#2860,#439,.T.);
#3398=EDGE_CURVE('',#2861,#2862,#1626,.T.);
#3399=EDGE_CURVE('',#2862,#2862,#2652,.T.);
#3400=EDGE_CURVE('',#2863,#2861,#440,.T.);
#3401=EDGE_CURVE('',#2860,#2863,#441,.T.);
#3402=EDGE_CURVE('',#2864,#2864,#2653,.T.);
#3403=EDGE_CURVE('',#2864,#2865,#1627,.T.);
#3404=EDGE_CURVE('',#2866,#2865,#442,.T.);
#3405=EDGE_CURVE('',#2866,#2867,#1628,.T.);
#3406=EDGE_CURVE('',#2867,#2867,#2654,.T.);
#3407=EDGE_CURVE('',#2868,#2866,#443,.T.);
#3408=EDGE_CURVE('',#2865,#2868,#444,.T.);
#3409=EDGE_CURVE('',#2869,#2870,#445,.T.);
#3410=EDGE_CURVE('',#2870,#2869,#446,.T.);
#3411=EDGE_CURVE('',#2856,#2866,#1629,.T.);
#3412=EDGE_CURVE('',#2871,#2871,#2655,.T.);
#3413=EDGE_CURVE('',#2871,#2861,#1630,.T.);
#3414=EDGE_CURVE('',#2872,#2873,#1631,.T.);
#3415=EDGE_CURVE('',#2872,#2874,#1632,.T.);
#3416=EDGE_CURVE('',#2875,#2874,#1633,.T.);
#3417=EDGE_CURVE('',#2873,#2875,#1634,.T.);
#3418=EDGE_CURVE('',#2876,#2872,#1635,.T.);
#3419=EDGE_CURVE('',#2876,#2877,#1636,.T.);
#3420=EDGE_CURVE('',#2874,#2877,#1637,.T.);
#3421=EDGE_CURVE('',#2878,#2876,#1638,.T.);
#3422=EDGE_CURVE('',#2878,#2879,#1639,.T.);
#3423=EDGE_CURVE('',#2877,#2879,#1640,.T.);
#3424=EDGE_CURVE('',#2880,#2878,#1641,.T.);
#3425=EDGE_CURVE('',#2880,#2881,#1642,.T.);
#3426=EDGE_CURVE('',#2879,#2881,#1643,.T.);
#3427=EDGE_CURVE('',#2882,#2880,#1644,.T.);
#3428=EDGE_CURVE('',#2882,#2883,#1645,.T.);
#3429=EDGE_CURVE('',#2881,#2883,#1646,.T.);
#3430=EDGE_CURVE('',#2884,#2882,#1647,.T.);
#3431=EDGE_CURVE('',#2884,#2885,#1648,.T.);
#3432=EDGE_CURVE('',#2883,#2885,#1649,.T.);
#3433=EDGE_CURVE('',#2886,#2884,#1650,.T.);
#3434=EDGE_CURVE('',#2886,#2887,#1651,.T.);
#3435=EDGE_CURVE('',#2885,#2887,#1652,.T.);
#3436=EDGE_CURVE('',#2888,#2886,#1653,.T.);
#3437=EDGE_CURVE('',#2888,#2889,#1654,.T.);
#3438=EDGE_CURVE('',#2887,#2889,#1655,.T.);
#3439=EDGE_CURVE('',#2890,#2888,#1656,.T.);
#3440=EDGE_CURVE('',#2891,#2890,#1657,.T.);
#3441=EDGE_CURVE('',#2889,#2891,#1658,.T.);
#3442=EDGE_CURVE('',#2892,#2893,#1659,.T.);
#3443=EDGE_CURVE('',#2892,#2894,#1660,.T.);
#3444=EDGE_CURVE('',#2895,#2894,#1661,.T.);
#3445=EDGE_CURVE('',#2893,#2895,#1662,.T.);
#3446=EDGE_CURVE('',#2896,#2892,#1663,.T.);
#3447=EDGE_CURVE('',#2896,#2897,#1664,.T.);
#3448=EDGE_CURVE('',#2894,#2897,#1665,.T.);
#3449=EDGE_CURVE('',#2898,#2896,#1666,.T.);
#3450=EDGE_CURVE('',#2898,#2899,#1667,.T.);
#3451=EDGE_CURVE('',#2897,#2899,#1668,.T.);
#3452=EDGE_CURVE('',#2900,#2898,#1669,.T.);
#3453=EDGE_CURVE('',#2900,#2901,#1670,.T.);
#3454=EDGE_CURVE('',#2899,#2901,#1671,.T.);
#3455=EDGE_CURVE('',#2902,#2900,#1672,.T.);
#3456=EDGE_CURVE('',#2902,#2903,#1673,.T.);
#3457=EDGE_CURVE('',#2901,#2903,#1674,.T.);
#3458=EDGE_CURVE('',#2904,#2902,#1675,.T.);
#3459=EDGE_CURVE('',#2904,#2905,#1676,.T.);
#3460=EDGE_CURVE('',#2903,#2905,#1677,.T.);
#3461=EDGE_CURVE('',#2906,#2904,#1678,.T.);
#3462=EDGE_CURVE('',#2906,#2907,#1679,.T.);
#3463=EDGE_CURVE('',#2905,#2907,#1680,.T.);
#3464=EDGE_CURVE('',#2908,#2906,#1681,.T.);
#3465=EDGE_CURVE('',#2908,#2909,#1682,.T.);
#3466=EDGE_CURVE('',#2907,#2909,#1683,.T.);
#3467=EDGE_CURVE('',#2910,#2908,#1684,.T.);
#3468=EDGE_CURVE('',#2911,#2910,#1685,.T.);
#3469=EDGE_CURVE('',#2909,#2911,#1686,.T.);
#3470=EDGE_CURVE('',#2912,#2913,#1687,.T.);
#3471=EDGE_CURVE('',#2912,#2914,#1688,.T.);
#3472=EDGE_CURVE('',#2915,#2914,#1689,.T.);
#3473=EDGE_CURVE('',#2913,#2915,#1690,.T.);
#3474=EDGE_CURVE('',#2916,#2912,#1691,.T.);
#3475=EDGE_CURVE('',#2916,#2917,#1692,.T.);
#3476=EDGE_CURVE('',#2914,#2917,#1693,.T.);
#3477=EDGE_CURVE('',#2918,#2916,#1694,.T.);
#3478=EDGE_CURVE('',#2918,#2919,#1695,.T.);
#3479=EDGE_CURVE('',#2917,#2919,#1696,.T.);
#3480=EDGE_CURVE('',#2920,#2918,#1697,.T.);
#3481=EDGE_CURVE('',#2920,#2921,#1698,.T.);
#3482=EDGE_CURVE('',#2919,#2921,#1699,.T.);
#3483=EDGE_CURVE('',#2922,#2920,#1700,.T.);
#3484=EDGE_CURVE('',#2922,#2923,#1701,.T.);
#3485=EDGE_CURVE('',#2921,#2923,#1702,.T.);
#3486=EDGE_CURVE('',#2924,#2922,#1703,.T.);
#3487=EDGE_CURVE('',#2924,#2925,#1704,.T.);
#3488=EDGE_CURVE('',#2923,#2925,#1705,.T.);
#3489=EDGE_CURVE('',#2926,#2924,#1706,.T.);
#3490=EDGE_CURVE('',#2926,#2927,#1707,.T.);
#3491=EDGE_CURVE('',#2925,#2927,#1708,.T.);
#3492=EDGE_CURVE('',#2928,#2926,#1709,.T.);
#3493=EDGE_CURVE('',#2928,#2929,#1710,.T.);
#3494=EDGE_CURVE('',#2927,#2929,#1711,.T.);
#3495=EDGE_CURVE('',#2930,#2928,#1712,.T.);
#3496=EDGE_CURVE('',#2931,#2930,#1713,.T.);
#3497=EDGE_CURVE('',#2929,#2931,#1714,.T.);
#3498=EDGE_CURVE('',#2932,#2933,#1715,.T.);
#3499=EDGE_CURVE('',#2932,#2934,#1716,.T.);
#3500=EDGE_CURVE('',#2935,#2934,#1717,.T.);
#3501=EDGE_CURVE('',#2933,#2935,#1718,.T.);
#3502=EDGE_CURVE('',#2936,#2932,#1719,.T.);
#3503=EDGE_CURVE('',#2936,#2937,#1720,.T.);
#3504=EDGE_CURVE('',#2934,#2937,#1721,.T.);
#3505=EDGE_CURVE('',#2938,#2936,#1722,.T.);
#3506=EDGE_CURVE('',#2938,#2939,#1723,.T.);
#3507=EDGE_CURVE('',#2937,#2939,#1724,.T.);
#3508=EDGE_CURVE('',#2940,#2938,#1725,.T.);
#3509=EDGE_CURVE('',#2940,#2941,#1726,.T.);
#3510=EDGE_CURVE('',#2939,#2941,#1727,.T.);
#3511=EDGE_CURVE('',#2942,#2940,#1728,.T.);
#3512=EDGE_CURVE('',#2942,#2943,#1729,.T.);
#3513=EDGE_CURVE('',#2941,#2943,#1730,.T.);
#3514=EDGE_CURVE('',#2944,#2942,#1731,.T.);
#3515=EDGE_CURVE('',#2944,#2945,#1732,.T.);
#3516=EDGE_CURVE('',#2943,#2945,#1733,.T.);
#3517=EDGE_CURVE('',#2946,#2944,#1734,.T.);
#3518=EDGE_CURVE('',#2946,#2947,#1735,.T.);
#3519=EDGE_CURVE('',#2945,#2947,#1736,.T.);
#3520=EDGE_CURVE('',#2948,#2946,#1737,.T.);
#3521=EDGE_CURVE('',#2948,#2949,#1738,.T.);
#3522=EDGE_CURVE('',#2947,#2949,#1739,.T.);
#3523=EDGE_CURVE('',#2950,#2948,#1740,.T.);
#3524=EDGE_CURVE('',#2951,#2950,#1741,.T.);
#3525=EDGE_CURVE('',#2949,#2951,#1742,.T.);
#3526=EDGE_CURVE('',#2870,#2952,#1743,.T.);
#3527=EDGE_CURVE('',#2952,#2952,#2656,.T.);
#3528=EDGE_CURVE('',#2890,#2953,#1744,.T.);
#3529=EDGE_CURVE('',#2953,#2954,#1745,.T.);
#3530=EDGE_CURVE('',#2891,#2954,#1746,.T.);
#3531=EDGE_CURVE('',#2955,#2875,#1747,.T.);
#3532=EDGE_CURVE('',#2956,#2955,#1748,.T.);
#3533=EDGE_CURVE('',#2956,#2873,#1749,.T.);
#3534=EDGE_CURVE('',#2910,#2956,#1750,.T.);
#3535=EDGE_CURVE('',#2911,#2955,#1751,.T.);
#3536=EDGE_CURVE('',#2957,#2895,#1752,.T.);
#3537=EDGE_CURVE('',#2958,#2957,#1753,.T.);
#3538=EDGE_CURVE('',#2958,#2893,#1754,.T.);
#3539=EDGE_CURVE('',#2930,#2958,#1755,.T.);
#3540=EDGE_CURVE('',#2931,#2957,#1756,.T.);
#3541=EDGE_CURVE('',#2959,#2915,#1757,.T.);
#3542=EDGE_CURVE('',#2960,#2959,#1758,.T.);
#3543=EDGE_CURVE('',#2960,#2913,#1759,.T.);
#3544=EDGE_CURVE('',#2950,#2960,#1760,.T.);
#3545=EDGE_CURVE('',#2951,#2959,#1761,.T.);
#3546=EDGE_CURVE('',#2954,#2935,#1762,.T.);
#3547=EDGE_CURVE('',#2953,#2933,#1763,.T.);
#4273=ORIENTED_EDGE('',*,*,#3371,.F.);
#4274=ORIENTED_EDGE('',*,*,#3372,.T.);
#4275=ORIENTED_EDGE('',*,*,#3373,.F.);
#4276=ORIENTED_EDGE('',*,*,#3374,.F.);
#4277=ORIENTED_EDGE('',*,*,#3375,.T.);
#4278=ORIENTED_EDGE('',*,*,#3376,.F.);
#4279=ORIENTED_EDGE('',*,*,#3375,.F.);
#4280=ORIENTED_EDGE('',*,*,#3377,.F.);
#4281=ORIENTED_EDGE('',*,*,#3378,.F.);
#4282=ORIENTED_EDGE('',*,*,#3372,.F.);
#4283=ORIENTED_EDGE('',*,*,#3379,.F.);
#4284=ORIENTED_EDGE('',*,*,#3380,.F.);
#4285=ORIENTED_EDGE('',*,*,#3381,.F.);
#4286=ORIENTED_EDGE('',*,*,#3382,.T.);
#4287=ORIENTED_EDGE('',*,*,#3383,.F.);
#4288=ORIENTED_EDGE('',*,*,#3384,.F.);
#4289=ORIENTED_EDGE('',*,*,#3385,.T.);
#4290=ORIENTED_EDGE('',*,*,#3386,.F.);
#4291=ORIENTED_EDGE('',*,*,#3385,.F.);
#4292=ORIENTED_EDGE('',*,*,#3387,.F.);
#4293=ORIENTED_EDGE('',*,*,#3388,.F.);
#4294=ORIENTED_EDGE('',*,*,#3382,.F.);
#4295=ORIENTED_EDGE('',*,*,#3389,.F.);
#4296=ORIENTED_EDGE('',*,*,#3390,.F.);
#4297=ORIENTED_EDGE('',*,*,#3379,.T.);
#4298=ORIENTED_EDGE('',*,*,#3391,.T.);
#4299=ORIENTED_EDGE('',*,*,#3383,.T.);
#4300=ORIENTED_EDGE('',*,*,#3388,.T.);
#4301=ORIENTED_EDGE('',*,*,#3387,.T.);
#4302=ORIENTED_EDGE('',*,*,#3384,.T.);
#4303=ORIENTED_EDGE('',*,*,#3391,.F.);
#4304=ORIENTED_EDGE('',*,*,#3380,.T.);
#4305=ORIENTED_EDGE('',*,*,#3392,.T.);
#4306=ORIENTED_EDGE('',*,*,#3393,.T.);
#4307=ORIENTED_EDGE('',*,*,#3373,.T.);
#4308=ORIENTED_EDGE('',*,*,#3378,.T.);
#4309=ORIENTED_EDGE('',*,*,#3377,.T.);
#4310=ORIENTED_EDGE('',*,*,#3374,.T.);
#4311=ORIENTED_EDGE('',*,*,#3393,.F.);
#4312=ORIENTED_EDGE('',*,*,#3394,.T.);
#4313=ORIENTED_EDGE('',*,*,#3395,.F.);
#4314=ORIENTED_EDGE('',*,*,#3396,.T.);
#4315=ORIENTED_EDGE('',*,*,#3397,.F.);
#4316=ORIENTED_EDGE('',*,*,#3398,.T.);
#4317=ORIENTED_EDGE('',*,*,#3399,.F.);
#4318=ORIENTED_EDGE('',*,*,#3398,.F.);
#4319=ORIENTED_EDGE('',*,*,#3400,.F.);
#4320=ORIENTED_EDGE('',*,*,#3401,.F.);
#4321=ORIENTED_EDGE('',*,*,#3396,.F.);
#4322=ORIENTED_EDGE('',*,*,#3392,.F.);
#4323=ORIENTED_EDGE('',*,*,#3394,.F.);
#4324=ORIENTED_EDGE('',*,*,#3402,.F.);
#4325=ORIENTED_EDGE('',*,*,#3403,.T.);
#4326=ORIENTED_EDGE('',*,*,#3404,.F.);
#4327=ORIENTED_EDGE('',*,*,#3405,.T.);
#4328=ORIENTED_EDGE('',*,*,#3406,.F.);
#4329=ORIENTED_EDGE('',*,*,#3405,.F.);
#4330=ORIENTED_EDGE('',*,*,#3407,.F.);
#4331=ORIENTED_EDGE('',*,*,#3408,.F.);
#4332=ORIENTED_EDGE('',*,*,#3403,.F.);
#4333=ORIENTED_EDGE('',*,*,#3409,.F.);
#4334=ORIENTED_EDGE('',*,*,#3410,.F.);
#4335=ORIENTED_EDGE('',*,*,#3389,.T.);
#4336=ORIENTED_EDGE('',*,*,#3411,.T.);
#4337=ORIENTED_EDGE('',*,*,#3404,.T.);
#4338=ORIENTED_EDGE('',*,*,#3408,.T.);
#4339=ORIENTED_EDGE('',*,*,#3407,.T.);
#4340=ORIENTED_EDGE('',*,*,#3411,.F.);
#4341=ORIENTED_EDGE('',*,*,#3390,.T.);
#4342=ORIENTED_EDGE('',*,*,#3412,.F.);
#4343=ORIENTED_EDGE('',*,*,#3413,.T.);
#4344=ORIENTED_EDGE('',*,*,#3397,.T.);
#4345=ORIENTED_EDGE('',*,*,#3401,.T.);
#4346=ORIENTED_EDGE('',*,*,#3400,.T.);
#4347=ORIENTED_EDGE('',*,*,#3413,.F.);
#4348=ORIENTED_EDGE('',*,*,#3414,.F.);
#4349=ORIENTED_EDGE('',*,*,#3415,.T.);
#4350=ORIENTED_EDGE('',*,*,#3416,.F.);
#4351=ORIENTED_EDGE('',*,*,#3417,.F.);
#4352=ORIENTED_EDGE('',*,*,#3418,.F.);
#4353=ORIENTED_EDGE('',*,*,#3419,.T.);
#4354=ORIENTED_EDGE('',*,*,#3420,.F.);
#4355=ORIENTED_EDGE('',*,*,#3415,.F.);
#4356=ORIENTED_EDGE('',*,*,#3421,.F.);
#4357=ORIENTED_EDGE('',*,*,#3422,.T.);
#4358=ORIENTED_EDGE('',*,*,#3423,.F.);
#4359=ORIENTED_EDGE('',*,*,#3419,.F.);
#4360=ORIENTED_EDGE('',*,*,#3424,.F.);
#4361=ORIENTED_EDGE('',*,*,#3425,.T.);
#4362=ORIENTED_EDGE('',*,*,#3426,.F.);
#4363=ORIENTED_EDGE('',*,*,#3422,.F.);
#4364=ORIENTED_EDGE('',*,*,#3427,.F.);
#4365=ORIENTED_EDGE('',*,*,#3428,.T.);
#4366=ORIENTED_EDGE('',*,*,#3429,.F.);
#4367=ORIENTED_EDGE('',*,*,#3425,.F.);
#4368=ORIENTED_EDGE('',*,*,#3376,.T.);
#4369=ORIENTED_EDGE('',*,*,#3386,.T.);
#4370=ORIENTED_EDGE('',*,*,#3430,.F.);
#4371=ORIENTED_EDGE('',*,*,#3431,.T.);
#4372=ORIENTED_EDGE('',*,*,#3432,.F.);
#4373=ORIENTED_EDGE('',*,*,#3428,.F.);
#4374=ORIENTED_EDGE('',*,*,#3433,.F.);
#4375=ORIENTED_EDGE('',*,*,#3434,.T.);
#4376=ORIENTED_EDGE('',*,*,#3435,.F.);
#4377=ORIENTED_EDGE('',*,*,#3431,.F.);
#4378=ORIENTED_EDGE('',*,*,#3436,.F.);
#4379=ORIENTED_EDGE('',*,*,#3437,.T.);
#4380=ORIENTED_EDGE('',*,*,#3438,.F.);
#4381=ORIENTED_EDGE('',*,*,#3434,.F.);
#4382=ORIENTED_EDGE('',*,*,#3439,.F.);
#4383=ORIENTED_EDGE('',*,*,#3440,.F.);
#4384=ORIENTED_EDGE('',*,*,#3441,.F.);
#4385=ORIENTED_EDGE('',*,*,#3437,.F.);
#4386=ORIENTED_EDGE('',*,*,#3442,.F.);
#4387=ORIENTED_EDGE('',*,*,#3443,.T.);
#4388=ORIENTED_EDGE('',*,*,#3444,.F.);
#4389=ORIENTED_EDGE('',*,*,#3445,.F.);
#4390=ORIENTED_EDGE('',*,*,#3446,.F.);
#4391=ORIENTED_EDGE('',*,*,#3447,.T.);
#4392=ORIENTED_EDGE('',*,*,#3448,.F.);
#4393=ORIENTED_EDGE('',*,*,#3443,.F.);
#4394=ORIENTED_EDGE('',*,*,#3449,.F.);
#4395=ORIENTED_EDGE('',*,*,#3450,.T.);
#4396=ORIENTED_EDGE('',*,*,#3451,.F.);
#4397=ORIENTED_EDGE('',*,*,#3447,.F.);
#4398=ORIENTED_EDGE('',*,*,#3452,.F.);
#4399=ORIENTED_EDGE('',*,*,#3453,.T.);
#4400=ORIENTED_EDGE('',*,*,#3454,.F.);
#4401=ORIENTED_EDGE('',*,*,#3450,.F.);
#4402=ORIENTED_EDGE('',*,*,#3455,.F.);
#4403=ORIENTED_EDGE('',*,*,#3456,.T.);
#4404=ORIENTED_EDGE('',*,*,#3457,.F.);
#4405=ORIENTED_EDGE('',*,*,#3453,.F.);
#4406=ORIENTED_EDGE('',*,*,#3395,.T.);
#4407=ORIENTED_EDGE('',*,*,#3402,.T.);
#4408=ORIENTED_EDGE('',*,*,#3458,.F.);
#4409=ORIENTED_EDGE('',*,*,#3459,.T.);
#4410=ORIENTED_EDGE('',*,*,#3460,.F.);
#4411=ORIENTED_EDGE('',*,*,#3456,.F.);
#4412=ORIENTED_EDGE('',*,*,#3461,.F.);
#4413=ORIENTED_EDGE('',*,*,#3462,.T.);
#4414=ORIENTED_EDGE('',*,*,#3463,.F.);
#4415=ORIENTED_EDGE('',*,*,#3459,.F.);
#4416=ORIENTED_EDGE('',*,*,#3464,.F.);
#4417=ORIENTED_EDGE('',*,*,#3465,.T.);
#4418=ORIENTED_EDGE('',*,*,#3466,.F.);
#4419=ORIENTED_EDGE('',*,*,#3462,.F.);
#4420=ORIENTED_EDGE('',*,*,#3467,.F.);
#4421=ORIENTED_EDGE('',*,*,#3468,.F.);
#4422=ORIENTED_EDGE('',*,*,#3469,.F.);
#4423=ORIENTED_EDGE('',*,*,#3465,.F.);
#4424=ORIENTED_EDGE('',*,*,#3470,.F.);
#4425=ORIENTED_EDGE('',*,*,#3471,.T.);
#4426=ORIENTED_EDGE('',*,*,#3472,.F.);
#4427=ORIENTED_EDGE('',*,*,#3473,.F.);
#4428=ORIENTED_EDGE('',*,*,#3474,.F.);
#4429=ORIENTED_EDGE('',*,*,#3475,.T.);
#4430=ORIENTED_EDGE('',*,*,#3476,.F.);
#4431=ORIENTED_EDGE('',*,*,#3471,.F.);
#4432=ORIENTED_EDGE('',*,*,#3477,.F.);
#4433=ORIENTED_EDGE('',*,*,#3478,.T.);
#4434=ORIENTED_EDGE('',*,*,#3479,.F.);
#4435=ORIENTED_EDGE('',*,*,#3475,.F.);
#4436=ORIENTED_EDGE('',*,*,#3480,.F.);
#4437=ORIENTED_EDGE('',*,*,#3481,.T.);
#4438=ORIENTED_EDGE('',*,*,#3482,.F.);
#4439=ORIENTED_EDGE('',*,*,#3478,.F.);
#4440=ORIENTED_EDGE('',*,*,#3483,.F.);
#4441=ORIENTED_EDGE('',*,*,#3484,.T.);
#4442=ORIENTED_EDGE('',*,*,#3485,.F.);
#4443=ORIENTED_EDGE('',*,*,#3481,.F.);
#4444=ORIENTED_EDGE('',*,*,#3371,.T.);
#4445=ORIENTED_EDGE('',*,*,#3381,.T.);
#4446=ORIENTED_EDGE('',*,*,#3486,.F.);
#4447=ORIENTED_EDGE('',*,*,#3487,.T.);
#4448=ORIENTED_EDGE('',*,*,#3488,.F.);
#4449=ORIENTED_EDGE('',*,*,#3484,.F.);
#4450=ORIENTED_EDGE('',*,*,#3489,.F.);
#4451=ORIENTED_EDGE('',*,*,#3490,.T.);
#4452=ORIENTED_EDGE('',*,*,#3491,.F.);
#4453=ORIENTED_EDGE('',*,*,#3487,.F.);
#4454=ORIENTED_EDGE('',*,*,#3492,.F.);
#4455=ORIENTED_EDGE('',*,*,#3493,.T.);
#4456=ORIENTED_EDGE('',*,*,#3494,.F.);
#4457=ORIENTED_EDGE('',*,*,#3490,.F.);
#4458=ORIENTED_EDGE('',*,*,#3495,.F.);
#4459=ORIENTED_EDGE('',*,*,#3496,.F.);
#4460=ORIENTED_EDGE('',*,*,#3497,.F.);
#4461=ORIENTED_EDGE('',*,*,#3493,.F.);
#4462=ORIENTED_EDGE('',*,*,#3498,.F.);
#4463=ORIENTED_EDGE('',*,*,#3499,.T.);
#4464=ORIENTED_EDGE('',*,*,#3500,.F.);
#4465=ORIENTED_EDGE('',*,*,#3501,.F.);
#4466=ORIENTED_EDGE('',*,*,#3502,.F.);
#4467=ORIENTED_EDGE('',*,*,#3503,.T.);
#4468=ORIENTED_EDGE('',*,*,#3504,.F.);
#4469=ORIENTED_EDGE('',*,*,#3499,.F.);
#4470=ORIENTED_EDGE('',*,*,#3505,.F.);
#4471=ORIENTED_EDGE('',*,*,#3506,.T.);
#4472=ORIENTED_EDGE('',*,*,#3507,.F.);
#4473=ORIENTED_EDGE('',*,*,#3503,.F.);
#4474=ORIENTED_EDGE('',*,*,#3508,.F.);
#4475=ORIENTED_EDGE('',*,*,#3509,.T.);
#4476=ORIENTED_EDGE('',*,*,#3510,.F.);
#4477=ORIENTED_EDGE('',*,*,#3506,.F.);
#4478=ORIENTED_EDGE('',*,*,#3511,.F.);
#4479=ORIENTED_EDGE('',*,*,#3512,.T.);
#4480=ORIENTED_EDGE('',*,*,#3513,.F.);
#4481=ORIENTED_EDGE('',*,*,#3509,.F.);
#4482=ORIENTED_EDGE('',*,*,#3399,.T.);
#4483=ORIENTED_EDGE('',*,*,#3406,.T.);
#4484=ORIENTED_EDGE('',*,*,#3514,.F.);
#4485=ORIENTED_EDGE('',*,*,#3515,.T.);
#4486=ORIENTED_EDGE('',*,*,#3516,.F.);
#4487=ORIENTED_EDGE('',*,*,#3512,.F.);
#4488=ORIENTED_EDGE('',*,*,#3517,.F.);
#4489=ORIENTED_EDGE('',*,*,#3518,.T.);
#4490=ORIENTED_EDGE('',*,*,#3519,.F.);
#4491=ORIENTED_EDGE('',*,*,#3515,.F.);
#4492=ORIENTED_EDGE('',*,*,#3520,.F.);
#4493=ORIENTED_EDGE('',*,*,#3521,.T.);
#4494=ORIENTED_EDGE('',*,*,#3522,.F.);
#4495=ORIENTED_EDGE('',*,*,#3518,.F.);
#4496=ORIENTED_EDGE('',*,*,#3523,.F.);
#4497=ORIENTED_EDGE('',*,*,#3524,.F.);
#4498=ORIENTED_EDGE('',*,*,#3525,.F.);
#4499=ORIENTED_EDGE('',*,*,#3521,.F.);
#4500=ORIENTED_EDGE('',*,*,#3409,.T.);
#4501=ORIENTED_EDGE('',*,*,#3526,.T.);
#4502=ORIENTED_EDGE('',*,*,#3527,.F.);
#4503=ORIENTED_EDGE('',*,*,#3526,.F.);
#4504=ORIENTED_EDGE('',*,*,#3410,.T.);
#4505=ORIENTED_EDGE('',*,*,#3440,.T.);
#4506=ORIENTED_EDGE('',*,*,#3528,.T.);
#4507=ORIENTED_EDGE('',*,*,#3529,.T.);
#4508=ORIENTED_EDGE('',*,*,#3530,.F.);
#4509=ORIENTED_EDGE('',*,*,#3417,.T.);
#4510=ORIENTED_EDGE('',*,*,#3531,.F.);
#4511=ORIENTED_EDGE('',*,*,#3532,.F.);
#4512=ORIENTED_EDGE('',*,*,#3533,.T.);
#4513=ORIENTED_EDGE('',*,*,#3468,.T.);
#4514=ORIENTED_EDGE('',*,*,#3534,.T.);
#4515=ORIENTED_EDGE('',*,*,#3532,.T.);
#4516=ORIENTED_EDGE('',*,*,#3535,.F.);
#4517=ORIENTED_EDGE('',*,*,#3445,.T.);
#4518=ORIENTED_EDGE('',*,*,#3536,.F.);
#4519=ORIENTED_EDGE('',*,*,#3537,.F.);
#4520=ORIENTED_EDGE('',*,*,#3538,.T.);
#4521=ORIENTED_EDGE('',*,*,#3496,.T.);
#4522=ORIENTED_EDGE('',*,*,#3539,.T.);
#4523=ORIENTED_EDGE('',*,*,#3537,.T.);
#4524=ORIENTED_EDGE('',*,*,#3540,.F.);
#4525=ORIENTED_EDGE('',*,*,#3473,.T.);
#4526=ORIENTED_EDGE('',*,*,#3541,.F.);
#4527=ORIENTED_EDGE('',*,*,#3542,.F.);
#4528=ORIENTED_EDGE('',*,*,#3543,.T.);
#4529=ORIENTED_EDGE('',*,*,#3524,.T.);
#4530=ORIENTED_EDGE('',*,*,#3544,.T.);
#4531=ORIENTED_EDGE('',*,*,#3542,.T.);
#4532=ORIENTED_EDGE('',*,*,#3545,.F.);
#4533=ORIENTED_EDGE('',*,*,#3501,.T.);
#4534=ORIENTED_EDGE('',*,*,#3546,.F.);
#4535=ORIENTED_EDGE('',*,*,#3529,.F.);
#4536=ORIENTED_EDGE('',*,*,#3547,.T.);
#4537=ORIENTED_EDGE('',*,*,#3416,.T.);
#4538=ORIENTED_EDGE('',*,*,#3420,.T.);
#4539=ORIENTED_EDGE('',*,*,#3423,.T.);
#4540=ORIENTED_EDGE('',*,*,#3426,.T.);
#4541=ORIENTED_EDGE('',*,*,#3429,.T.);
#4542=ORIENTED_EDGE('',*,*,#3432,.T.);
#4543=ORIENTED_EDGE('',*,*,#3435,.T.);
#4544=ORIENTED_EDGE('',*,*,#3438,.T.);
#4545=ORIENTED_EDGE('',*,*,#3441,.T.);
#4546=ORIENTED_EDGE('',*,*,#3530,.T.);
#4547=ORIENTED_EDGE('',*,*,#3546,.T.);
#4548=ORIENTED_EDGE('',*,*,#3500,.T.);
#4549=ORIENTED_EDGE('',*,*,#3504,.T.);
#4550=ORIENTED_EDGE('',*,*,#3507,.T.);
#4551=ORIENTED_EDGE('',*,*,#3510,.T.);
#4552=ORIENTED_EDGE('',*,*,#3513,.T.);
#4553=ORIENTED_EDGE('',*,*,#3516,.T.);
#4554=ORIENTED_EDGE('',*,*,#3519,.T.);
#4555=ORIENTED_EDGE('',*,*,#3522,.T.);
#4556=ORIENTED_EDGE('',*,*,#3525,.T.);
#4557=ORIENTED_EDGE('',*,*,#3545,.T.);
#4558=ORIENTED_EDGE('',*,*,#3541,.T.);
#4559=ORIENTED_EDGE('',*,*,#3472,.T.);
#4560=ORIENTED_EDGE('',*,*,#3476,.T.);
#4561=ORIENTED_EDGE('',*,*,#3479,.T.);
#4562=ORIENTED_EDGE('',*,*,#3482,.T.);
#4563=ORIENTED_EDGE('',*,*,#3485,.T.);
#4564=ORIENTED_EDGE('',*,*,#3488,.T.);
#4565=ORIENTED_EDGE('',*,*,#3491,.T.);
#4566=ORIENTED_EDGE('',*,*,#3494,.T.);
#4567=ORIENTED_EDGE('',*,*,#3497,.T.);
#4568=ORIENTED_EDGE('',*,*,#3540,.T.);
#4569=ORIENTED_EDGE('',*,*,#3536,.T.);
#4570=ORIENTED_EDGE('',*,*,#3444,.T.);
#4571=ORIENTED_EDGE('',*,*,#3448,.T.);
#4572=ORIENTED_EDGE('',*,*,#3451,.T.);
#4573=ORIENTED_EDGE('',*,*,#3454,.T.);
#4574=ORIENTED_EDGE('',*,*,#3457,.T.);
#4575=ORIENTED_EDGE('',*,*,#3460,.T.);
#4576=ORIENTED_EDGE('',*,*,#3463,.T.);
#4577=ORIENTED_EDGE('',*,*,#3466,.T.);
#4578=ORIENTED_EDGE('',*,*,#3469,.T.);
#4579=ORIENTED_EDGE('',*,*,#3535,.T.);
#4580=ORIENTED_EDGE('',*,*,#3531,.T.);
#4581=ORIENTED_EDGE('',*,*,#3527,.T.);
#4582=ORIENTED_EDGE('',*,*,#3414,.T.);
#4583=ORIENTED_EDGE('',*,*,#3533,.F.);
#4584=ORIENTED_EDGE('',*,*,#3534,.F.);
#4585=ORIENTED_EDGE('',*,*,#3467,.T.);
#4586=ORIENTED_EDGE('',*,*,#3464,.T.);
#4587=ORIENTED_EDGE('',*,*,#3461,.T.);
#4588=ORIENTED_EDGE('',*,*,#3458,.T.);
#4589=ORIENTED_EDGE('',*,*,#3455,.T.);
#4590=ORIENTED_EDGE('',*,*,#3452,.T.);
#4591=ORIENTED_EDGE('',*,*,#3449,.T.);
#4592=ORIENTED_EDGE('',*,*,#3446,.T.);
#4593=ORIENTED_EDGE('',*,*,#3442,.T.);
#4594=ORIENTED_EDGE('',*,*,#3538,.F.);
#4595=ORIENTED_EDGE('',*,*,#3539,.F.);
#4596=ORIENTED_EDGE('',*,*,#3495,.T.);
#4597=ORIENTED_EDGE('',*,*,#3492,.T.);
#4598=ORIENTED_EDGE('',*,*,#3489,.T.);
#4599=ORIENTED_EDGE('',*,*,#3486,.T.);
#4600=ORIENTED_EDGE('',*,*,#3483,.T.);
#4601=ORIENTED_EDGE('',*,*,#3480,.T.);
#4602=ORIENTED_EDGE('',*,*,#3477,.T.);
#4603=ORIENTED_EDGE('',*,*,#3474,.T.);
#4604=ORIENTED_EDGE('',*,*,#3470,.T.);
#4605=ORIENTED_EDGE('',*,*,#3543,.F.);
#4606=ORIENTED_EDGE('',*,*,#3544,.F.);
#4607=ORIENTED_EDGE('',*,*,#3523,.T.);
#4608=ORIENTED_EDGE('',*,*,#3520,.T.);
#4609=ORIENTED_EDGE('',*,*,#3517,.T.);
#4610=ORIENTED_EDGE('',*,*,#3514,.T.);
#4611=ORIENTED_EDGE('',*,*,#3511,.T.);
#4612=ORIENTED_EDGE('',*,*,#3508,.T.);
#4613=ORIENTED_EDGE('',*,*,#3505,.T.);
#4614=ORIENTED_EDGE('',*,*,#3502,.T.);
#4615=ORIENTED_EDGE('',*,*,#3498,.T.);
#4616=ORIENTED_EDGE('',*,*,#3547,.F.);
#4617=ORIENTED_EDGE('',*,*,#3528,.F.);
#4618=ORIENTED_EDGE('',*,*,#3439,.T.);
#4619=ORIENTED_EDGE('',*,*,#3436,.T.);
#4620=ORIENTED_EDGE('',*,*,#3433,.T.);
#4621=ORIENTED_EDGE('',*,*,#3430,.T.);
#4622=ORIENTED_EDGE('',*,*,#3427,.T.);
#4623=ORIENTED_EDGE('',*,*,#3424,.T.);
#4624=ORIENTED_EDGE('',*,*,#3421,.T.);
#4625=ORIENTED_EDGE('',*,*,#3418,.T.);
#4626=ORIENTED_EDGE('',*,*,#3412,.T.);
#5297=CYLINDRICAL_SURFACE('',#6067,0.275);
#5298=CYLINDRICAL_SURFACE('',#6070,0.274999999999999);
#5299=CYLINDRICAL_SURFACE('',#6073,0.21);
#5300=CYLINDRICAL_SURFACE('',#6074,0.21);
#5301=CYLINDRICAL_SURFACE('',#6075,0.275);
#5302=CYLINDRICAL_SURFACE('',#6078,0.274999999999999);
#5303=CYLINDRICAL_SURFACE('',#6081,0.21);
#5304=CYLINDRICAL_SURFACE('',#6082,0.21);
#5305=CYLINDRICAL_SURFACE('',#6120,0.21);
#5419=ADVANCED_FACE('',(#923,#583),#5297,.F.);
#5420=ADVANCED_FACE('',(#924,#584),#5298,.F.);
#5421=ADVANCED_FACE('',(#925),#5299,.F.);
#5422=ADVANCED_FACE('',(#926),#5300,.F.);
#5423=ADVANCED_FACE('',(#927,#585),#5301,.F.);
#5424=ADVANCED_FACE('',(#928,#586),#5302,.F.);
#5425=ADVANCED_FACE('',(#929),#5303,.F.);
#5426=ADVANCED_FACE('',(#930),#5304,.F.);
#5427=ADVANCED_FACE('',(#931),#671,.F.);
#5428=ADVANCED_FACE('',(#932),#672,.F.);
#5429=ADVANCED_FACE('',(#933),#673,.F.);
#5430=ADVANCED_FACE('',(#934),#674,.F.);
#5431=ADVANCED_FACE('',(#935,#587,#588),#675,.F.);
#5432=ADVANCED_FACE('',(#936),#676,.F.);
#5433=ADVANCED_FACE('',(#937),#677,.F.);
#5434=ADVANCED_FACE('',(#938),#678,.F.);
#5435=ADVANCED_FACE('',(#939),#679,.F.);
#5436=ADVANCED_FACE('',(#940),#680,.F.);
#5437=ADVANCED_FACE('',(#941),#681,.F.);
#5438=ADVANCED_FACE('',(#942),#682,.F.);
#5439=ADVANCED_FACE('',(#943),#683,.F.);
#5440=ADVANCED_FACE('',(#944,#589,#590),#684,.F.);
#5441=ADVANCED_FACE('',(#945),#685,.F.);
#5442=ADVANCED_FACE('',(#946),#686,.F.);
#5443=ADVANCED_FACE('',(#947),#687,.F.);
#5444=ADVANCED_FACE('',(#948),#688,.F.);
#5445=ADVANCED_FACE('',(#949),#689,.F.);
#5446=ADVANCED_FACE('',(#950),#690,.F.);
#5447=ADVANCED_FACE('',(#951),#691,.F.);
#5448=ADVANCED_FACE('',(#952),#692,.F.);
#5449=ADVANCED_FACE('',(#953,#591,#592),#693,.F.);
#5450=ADVANCED_FACE('',(#954),#694,.F.);
#5451=ADVANCED_FACE('',(#955),#695,.F.);
#5452=ADVANCED_FACE('',(#956),#696,.F.);
#5453=ADVANCED_FACE('',(#957),#697,.F.);
#5454=ADVANCED_FACE('',(#958),#698,.F.);
#5455=ADVANCED_FACE('',(#959),#699,.F.);
#5456=ADVANCED_FACE('',(#960),#700,.F.);
#5457=ADVANCED_FACE('',(#961),#701,.F.);
#5458=ADVANCED_FACE('',(#962,#593,#594),#702,.F.);
#5459=ADVANCED_FACE('',(#963),#703,.F.);
#5460=ADVANCED_FACE('',(#964),#704,.F.);
#5461=ADVANCED_FACE('',(#965),#705,.F.);
#5462=ADVANCED_FACE('',(#966),#706,.F.);
#5463=ADVANCED_FACE('',(#967),#5305,.F.);
#5464=ADVANCED_FACE('',(#968),#707,.T.);
#5465=ADVANCED_FACE('',(#969),#708,.T.);
#5466=ADVANCED_FACE('',(#970),#709,.T.);
#5467=ADVANCED_FACE('',(#971),#710,.T.);
#5468=ADVANCED_FACE('',(#972),#711,.T.);
#5469=ADVANCED_FACE('',(#973),#712,.T.);
#5470=ADVANCED_FACE('',(#974),#713,.T.);
#5471=ADVANCED_FACE('',(#975),#714,.T.);
#5472=ADVANCED_FACE('',(#976,#595),#715,.T.);
#5473=ADVANCED_FACE('',(#977,#596),#716,.F.);
#5626=CLOSED_SHELL('',(#5419,#5420,#5421,#5422,#5423,#5424,#5425,#5426,
#5427,#5428,#5429,#5430,#5431,#5432,#5433,#5434,#5435,#5436,#5437,#5438,
#5439,#5440,#5441,#5442,#5443,#5444,#5445,#5446,#5447,#5448,#5449,#5450,
#5451,#5452,#5453,#5454,#5455,#5456,#5457,#5458,#5459,#5460,#5461,#5462,
#5463,#5464,#5465,#5466,#5467,#5468,#5469,#5470,#5471,#5472,#5473));
#6066=AXIS2_PLACEMENT_3D('',#8510,#6926,#6927);
#6067=AXIS2_PLACEMENT_3D('',#8511,#6928,#6929);
#6068=AXIS2_PLACEMENT_3D('',#8513,#6930,#6931);
#6069=AXIS2_PLACEMENT_3D('',#8544,#6934,#6935);
#6070=AXIS2_PLACEMENT_3D('',#8616,#6936,#6937);
#6071=AXIS2_PLACEMENT_3D('',#8618,#6938,#6939);
#6072=AXIS2_PLACEMENT_3D('',#8649,#6942,#6943);
#6073=AXIS2_PLACEMENT_3D('',#8721,#6944,#6945);
#6074=AXIS2_PLACEMENT_3D('',#8723,#6947,#6948);
#6075=AXIS2_PLACEMENT_3D('',#8771,#6950,#6951);
#6076=AXIS2_PLACEMENT_3D('',#8773,#6952,#6953);
#6077=AXIS2_PLACEMENT_3D('',#8801,#6956,#6957);
#6078=AXIS2_PLACEMENT_3D('',#8827,#6958,#6959);
#6079=AXIS2_PLACEMENT_3D('',#8829,#6960,#6961);
#6080=AXIS2_PLACEMENT_3D('',#8857,#6964,#6965);
#6081=AXIS2_PLACEMENT_3D('',#8929,#6966,#6967);
#6082=AXIS2_PLACEMENT_3D('',#8931,#6969,#6970);
#6083=AXIS2_PLACEMENT_3D('',#8933,#6971,#6972);
#6084=AXIS2_PLACEMENT_3D('',#8935,#6974,#6975);
#6085=AXIS2_PLACEMENT_3D('',#8944,#6980,#6981);
#6086=AXIS2_PLACEMENT_3D('',#8950,#6985,#6986);
#6087=AXIS2_PLACEMENT_3D('',#8956,#6990,#6991);
#6088=AXIS2_PLACEMENT_3D('',#8962,#6995,#6996);
#6089=AXIS2_PLACEMENT_3D('',#8968,#7000,#7001);
#6090=AXIS2_PLACEMENT_3D('',#8974,#7005,#7006);
#6091=AXIS2_PLACEMENT_3D('',#8980,#7010,#7011);
#6092=AXIS2_PLACEMENT_3D('',#8986,#7015,#7016);
#6093=AXIS2_PLACEMENT_3D('',#8992,#7020,#7021);
#6094=AXIS2_PLACEMENT_3D('',#9001,#7026,#7027);
#6095=AXIS2_PLACEMENT_3D('',#9007,#7031,#7032);
#6096=AXIS2_PLACEMENT_3D('',#9013,#7036,#7037);
#6097=AXIS2_PLACEMENT_3D('',#9019,#7041,#7042);
#6098=AXIS2_PLACEMENT_3D('',#9025,#7046,#7047);
#6099=AXIS2_PLACEMENT_3D('',#9031,#7051,#7052);
#6100=AXIS2_PLACEMENT_3D('',#9037,#7056,#7057);
#6101=AXIS2_PLACEMENT_3D('',#9043,#7061,#7062);
#6102=AXIS2_PLACEMENT_3D('',#9049,#7066,#7067);
#6103=AXIS2_PLACEMENT_3D('',#9058,#7072,#7073);
#6104=AXIS2_PLACEMENT_3D('',#9064,#7077,#7078);
#6105=AXIS2_PLACEMENT_3D('',#9070,#7082,#7083);
#6106=AXIS2_PLACEMENT_3D('',#9076,#7087,#7088);
#6107=AXIS2_PLACEMENT_3D('',#9082,#7092,#7093);
#6108=AXIS2_PLACEMENT_3D('',#9088,#7097,#7098);
#6109=AXIS2_PLACEMENT_3D('',#9094,#7102,#7103);
#6110=AXIS2_PLACEMENT_3D('',#9100,#7107,#7108);
#6111=AXIS2_PLACEMENT_3D('',#9106,#7112,#7113);
#6112=AXIS2_PLACEMENT_3D('',#9115,#7118,#7119);
#6113=AXIS2_PLACEMENT_3D('',#9121,#7123,#7124);
#6114=AXIS2_PLACEMENT_3D('',#9127,#7128,#7129);
#6115=AXIS2_PLACEMENT_3D('',#9133,#7133,#7134);
#6116=AXIS2_PLACEMENT_3D('',#9139,#7138,#7139);
#6117=AXIS2_PLACEMENT_3D('',#9145,#7143,#7144);
#6118=AXIS2_PLACEMENT_3D('',#9151,#7148,#7149);
#6119=AXIS2_PLACEMENT_3D('',#9157,#7153,#7154);
#6120=AXIS2_PLACEMENT_3D('',#9163,#7158,#7159);
#6121=AXIS2_PLACEMENT_3D('',#9166,#7161,#7162);
#6122=AXIS2_PLACEMENT_3D('',#9167,#7163,#7164);
#6123=AXIS2_PLACEMENT_3D('',#9173,#7168,#7169);
#6124=AXIS2_PLACEMENT_3D('',#9179,#7173,#7174);
#6125=AXIS2_PLACEMENT_3D('',#9182,#7177,#7178);
#6126=AXIS2_PLACEMENT_3D('',#9188,#7182,#7183);
#6127=AXIS2_PLACEMENT_3D('',#9191,#7186,#7187);
#6128=AXIS2_PLACEMENT_3D('',#9197,#7191,#7192);
#6129=AXIS2_PLACEMENT_3D('',#9200,#7195,#7196);
#6130=AXIS2_PLACEMENT_3D('',#9203,#7199,#7200);
#6131=AXIS2_PLACEMENT_3D('',#9204,#7201,#7202);
#6926=DIRECTION('axis',(0.,0.,1.));
#6927=DIRECTION('refdir',(1.,0.,0.));
#6928=DIRECTION('center_axis',(0.,1.,0.));
#6929=DIRECTION('ref_axis',(1.,0.,0.));
#6930=DIRECTION('center_axis',(0.,1.,0.));
#6931=DIRECTION('ref_axis',(1.,0.,0.));
#6932=DIRECTION('',(0.,1.,0.));
#6933=DIRECTION('',(0.,1.,0.));
#6934=DIRECTION('center_axis',(0.,-1.,2.77555756156289E-16));
#6935=DIRECTION('ref_axis',(1.,0.,0.));
#6936=DIRECTION('center_axis',(0.,1.,0.));
#6937=DIRECTION('ref_axis',(1.,0.,0.));
#6938=DIRECTION('center_axis',(0.,1.,0.));
#6939=DIRECTION('ref_axis',(1.,0.,0.));
#6940=DIRECTION('',(0.,1.,0.));
#6941=DIRECTION('',(0.,1.,0.));
#6942=DIRECTION('center_axis',(0.,-1.,2.77555756156289E-16));
#6943=DIRECTION('ref_axis',(1.,0.,0.));
#6944=DIRECTION('center_axis',(1.,0.,0.));
#6945=DIRECTION('ref_axis',(0.,0.,-1.));
#6946=DIRECTION('',(1.,0.,0.));
#6947=DIRECTION('center_axis',(1.,0.,0.));
#6948=DIRECTION('ref_axis',(0.,0.,-1.));
#6949=DIRECTION('',(1.,0.,0.));
#6950=DIRECTION('center_axis',(0.,0.,1.));
#6951=DIRECTION('ref_axis',(1.,0.,0.));
#6952=DIRECTION('center_axis',(0.,0.,1.));
#6953=DIRECTION('ref_axis',(1.,0.,0.));
#6954=DIRECTION('',(0.,0.,1.));
#6955=DIRECTION('',(0.,0.,1.));
#6956=DIRECTION('center_axis',(0.,0.,-1.));
#6957=DIRECTION('ref_axis',(1.,0.,0.));
#6958=DIRECTION('center_axis',(0.,0.,1.));
#6959=DIRECTION('ref_axis',(1.,0.,0.));
#6960=DIRECTION('center_axis',(0.,0.,1.));
#6961=DIRECTION('ref_axis',(1.,0.,0.));
#6962=DIRECTION('',(0.,0.,1.));
#6963=DIRECTION('',(0.,0.,1.));
#6964=DIRECTION('center_axis',(0.,0.,-1.));
#6965=DIRECTION('ref_axis',(1.,0.,0.));
#6966=DIRECTION('center_axis',(1.,0.,0.));
#6967=DIRECTION('ref_axis',(0.,0.,-1.));
#6968=DIRECTION('',(1.,0.,0.));
#6969=DIRECTION('center_axis',(1.,0.,0.));
#6970=DIRECTION('ref_axis',(0.,0.,-1.));
#6971=DIRECTION('center_axis',(1.,0.,0.));
#6972=DIRECTION('ref_axis',(0.,0.,-1.));
#6973=DIRECTION('',(1.,0.,0.));
#6974=DIRECTION('center_axis',(0.,0.,-1.));
#6975=DIRECTION('ref_axis',(0.,1.,0.));
#6976=DIRECTION('',(0.,1.,0.));
#6977=DIRECTION('',(1.,0.,0.));
#6978=DIRECTION('',(0.,-1.,0.));
#6979=DIRECTION('',(1.,0.,0.));
#6980=DIRECTION('center_axis',(0.,1.,-8.88178419700125E-16));
#6981=DIRECTION('ref_axis',(0.,8.88178419700125E-16,1.));
#6982=DIRECTION('',(0.,8.88178419700125E-16,1.));
#6983=DIRECTION('',(1.,0.,0.));
#6984=DIRECTION('',(0.,-8.88178419700125E-16,-1.));
#6985=DIRECTION('center_axis',(0.,-7.40148683083439E-16,-1.));
#6986=DIRECTION('ref_axis',(0.,1.,-7.40148683083439E-16));
#6987=DIRECTION('',(0.,1.,-7.40148683083439E-16));
#6988=DIRECTION('',(1.,0.,0.));
#6989=DIRECTION('',(0.,-1.,7.40148683083439E-16));
#6990=DIRECTION('center_axis',(0.,-0.707106781186547,-0.707106781186548));
#6991=DIRECTION('ref_axis',(0.,0.707106781186548,-0.707106781186547));
#6992=DIRECTION('',(0.,0.707106781186548,-0.707106781186547));
#6993=DIRECTION('',(1.,0.,0.));
#6994=DIRECTION('',(0.,-0.707106781186548,0.707106781186547));
#6995=DIRECTION('center_axis',(0.,-1.,2.77555756156289E-16));
#6996=DIRECTION('ref_axis',(0.,-2.77555756156289E-16,-1.));
#6997=DIRECTION('',(0.,-2.77555756156289E-16,-1.));
#6998=DIRECTION('',(1.,0.,0.));
#6999=DIRECTION('',(0.,2.77555756156289E-16,1.));
#7000=DIRECTION('center_axis',(0.,-0.707106781186547,0.707106781186548));
#7001=DIRECTION('ref_axis',(0.,-0.707106781186548,-0.707106781186547));
#7002=DIRECTION('',(0.,-0.707106781186548,-0.707106781186547));
#7003=DIRECTION('',(1.,0.,0.));
#7004=DIRECTION('',(0.,0.707106781186548,0.707106781186547));
#7005=DIRECTION('center_axis',(0.,7.40148683083438E-16,1.));
#7006=DIRECTION('ref_axis',(0.,-1.,7.40148683083438E-16));
#7007=DIRECTION('',(0.,-1.,7.40148683083438E-16));
#7008=DIRECTION('',(1.,0.,0.));
#7009=DIRECTION('',(0.,1.,-7.40148683083438E-16));
#7010=DIRECTION('center_axis',(0.,1.,-4.44089209850063E-16));
#7011=DIRECTION('ref_axis',(0.,4.44089209850063E-16,1.));
#7012=DIRECTION('',(0.,4.44089209850063E-16,1.));
#7013=DIRECTION('',(1.,0.,0.));
#7014=DIRECTION('',(0.,-4.44089209850063E-16,-1.));
#7015=DIRECTION('center_axis',(0.,2.41352831440251E-16,1.));
#7016=DIRECTION('ref_axis',(0.,-1.,2.41352831440251E-16));
#7017=DIRECTION('',(0.,-1.,2.41352831440251E-16));
#7018=DIRECTION('',(-1.,0.,0.));
#7019=DIRECTION('',(0.,1.,-2.41352831440251E-16));
#7020=DIRECTION('center_axis',(0.,-1.,2.41352831440251E-16));
#7021=DIRECTION('ref_axis',(0.,-2.41352831440251E-16,-1.));
#7022=DIRECTION('',(0.,-2.41352831440251E-16,-1.));
#7023=DIRECTION('',(1.,0.,0.));
#7024=DIRECTION('',(0.,2.41352831440251E-16,1.));
#7025=DIRECTION('',(1.,0.,0.));
#7026=DIRECTION('center_axis',(0.,0.,-1.));
#7027=DIRECTION('ref_axis',(0.,1.,0.));
#7028=DIRECTION('',(0.,1.,0.));
#7029=DIRECTION('',(1.,0.,0.));
#7030=DIRECTION('',(0.,-1.,0.));
#7031=DIRECTION('center_axis',(0.,-1.,0.));
#7032=DIRECTION('ref_axis',(0.,0.,-1.));
#7033=DIRECTION('',(0.,0.,-1.));
#7034=DIRECTION('',(1.,0.,0.));
#7035=DIRECTION('',(0.,0.,1.));
#7036=DIRECTION('center_axis',(0.,-0.707106781186547,0.707106781186548));
#7037=DIRECTION('ref_axis',(0.,-0.707106781186548,-0.707106781186547));
#7038=DIRECTION('',(0.,-0.707106781186548,-0.707106781186547));
#7039=DIRECTION('',(1.,0.,0.));
#7040=DIRECTION('',(0.,0.707106781186548,0.707106781186547));
#7041=DIRECTION('center_axis',(0.,0.,1.));
#7042=DIRECTION('ref_axis',(0.,-1.,0.));
#7043=DIRECTION('',(0.,-1.,0.));
#7044=DIRECTION('',(1.,0.,0.));
#7045=DIRECTION('',(0.,1.,0.));
#7046=DIRECTION('center_axis',(0.,0.707106781186548,0.707106781186547));
#7047=DIRECTION('ref_axis',(0.,-0.707106781186547,0.707106781186548));
#7048=DIRECTION('',(0.,-0.707106781186547,0.707106781186548));
#7049=DIRECTION('',(1.,0.,0.));
#7050=DIRECTION('',(0.,0.707106781186547,-0.707106781186548));
#7051=DIRECTION('center_axis',(0.,1.,0.));
#7052=DIRECTION('ref_axis',(0.,0.,1.));
#7053=DIRECTION('',(0.,0.,1.));
#7054=DIRECTION('',(1.,0.,0.));
#7055=DIRECTION('',(0.,0.,-1.));
#7056=DIRECTION('center_axis',(0.,0.,-1.));
#7057=DIRECTION('ref_axis',(0.,1.,0.));
#7058=DIRECTION('',(0.,1.,0.));
#7059=DIRECTION('',(1.,0.,0.));
#7060=DIRECTION('',(0.,-1.,0.));
#7061=DIRECTION('center_axis',(0.,1.,-2.41352831440251E-16));
#7062=DIRECTION('ref_axis',(0.,2.41352831440251E-16,1.));
#7063=DIRECTION('',(0.,2.41352831440251E-16,1.));
#7064=DIRECTION('',(-1.,0.,0.));
#7065=DIRECTION('',(0.,-2.41352831440251E-16,-1.));
#7066=DIRECTION('center_axis',(0.,0.,1.));
#7067=DIRECTION('ref_axis',(0.,-1.,0.));
#7068=DIRECTION('',(0.,-1.,0.));
#7069=DIRECTION('',(1.,0.,0.));
#7070=DIRECTION('',(0.,1.,0.));
#7071=DIRECTION('',(1.,0.,0.));
#7072=DIRECTION('center_axis',(0.,-1.,0.));
#7073=DIRECTION('ref_axis',(0.,0.,-1.));
#7074=DIRECTION('',(0.,0.,-1.));
#7075=DIRECTION('',(1.,0.,0.));
#7076=DIRECTION('',(0.,0.,1.));
#7077=DIRECTION('center_axis',(0.,0.,1.));
#7078=DIRECTION('ref_axis',(0.,-1.,0.));
#7079=DIRECTION('',(0.,-1.,0.));
#7080=DIRECTION('',(1.,0.,0.));
#7081=DIRECTION('',(0.,1.,0.));
#7082=DIRECTION('center_axis',(0.,0.707106781186548,0.707106781186548));
#7083=DIRECTION('ref_axis',(0.,-0.707106781186548,0.707106781186548));
#7084=DIRECTION('',(0.,-0.707106781186548,0.707106781186548));
#7085=DIRECTION('',(1.,0.,0.));
#7086=DIRECTION('',(0.,0.707106781186548,-0.707106781186548));
#7087=DIRECTION('center_axis',(0.,1.,0.));
#7088=DIRECTION('ref_axis',(0.,0.,1.));
#7089=DIRECTION('',(0.,0.,1.));
#7090=DIRECTION('',(1.,0.,0.));
#7091=DIRECTION('',(0.,0.,-1.));
#7092=DIRECTION('center_axis',(0.,0.707106781186548,-0.707106781186547));
#7093=DIRECTION('ref_axis',(0.,0.707106781186547,0.707106781186548));
#7094=DIRECTION('',(0.,0.707106781186547,0.707106781186548));
#7095=DIRECTION('',(1.,0.,0.));
#7096=DIRECTION('',(0.,-0.707106781186547,-0.707106781186548));
#7097=DIRECTION('center_axis',(0.,-7.40148683083438E-16,-1.));
#7098=DIRECTION('ref_axis',(0.,1.,-7.40148683083438E-16));
#7099=DIRECTION('',(0.,1.,-7.40148683083438E-16));
#7100=DIRECTION('',(1.,0.,0.));
#7101=DIRECTION('',(0.,-1.,7.40148683083438E-16));
#7102=DIRECTION('center_axis',(0.,-1.,0.));
#7103=DIRECTION('ref_axis',(0.,0.,-1.));
#7104=DIRECTION('',(0.,0.,-1.));
#7105=DIRECTION('',(1.,0.,0.));
#7106=DIRECTION('',(0.,0.,1.));
#7107=DIRECTION('center_axis',(0.,0.,-1.));
#7108=DIRECTION('ref_axis',(0.,1.,0.));
#7109=DIRECTION('',(0.,1.,0.));
#7110=DIRECTION('',(-1.,0.,0.));
#7111=DIRECTION('',(0.,-1.,0.));
#7112=DIRECTION('center_axis',(0.,1.,0.));
#7113=DIRECTION('ref_axis',(0.,0.,1.));
#7114=DIRECTION('',(0.,0.,1.));
#7115=DIRECTION('',(1.,0.,0.));
#7116=DIRECTION('',(0.,0.,-1.));
#7117=DIRECTION('',(1.,0.,0.));
#7118=DIRECTION('center_axis',(0.,0.,1.));
#7119=DIRECTION('ref_axis',(0.,-1.,0.));
#7120=DIRECTION('',(0.,-1.,0.));
#7121=DIRECTION('',(1.,0.,0.));
#7122=DIRECTION('',(0.,1.,0.));
#7123=DIRECTION('center_axis',(0.,1.,0.));
#7124=DIRECTION('ref_axis',(0.,0.,1.));
#7125=DIRECTION('',(0.,0.,1.));
#7126=DIRECTION('',(1.,0.,0.));
#7127=DIRECTION('',(0.,0.,-1.));
#7128=DIRECTION('center_axis',(0.,0.707106781186547,-0.707106781186548));
#7129=DIRECTION('ref_axis',(0.,0.707106781186548,0.707106781186547));
#7130=DIRECTION('',(0.,0.707106781186548,0.707106781186547));
#7131=DIRECTION('',(1.,0.,0.));
#7132=DIRECTION('',(0.,-0.707106781186548,-0.707106781186547));
#7133=DIRECTION('center_axis',(0.,0.,-1.));
#7134=DIRECTION('ref_axis',(0.,1.,0.));
#7135=DIRECTION('',(0.,1.,0.));
#7136=DIRECTION('',(1.,0.,0.));
#7137=DIRECTION('',(0.,-1.,0.));
#7138=DIRECTION('center_axis',(0.,-0.707106781186547,-0.707106781186548));
#7139=DIRECTION('ref_axis',(0.,0.707106781186548,-0.707106781186547));
#7140=DIRECTION('',(0.,0.707106781186548,-0.707106781186547));
#7141=DIRECTION('',(1.,0.,0.));
#7142=DIRECTION('',(0.,-0.707106781186548,0.707106781186547));
#7143=DIRECTION('center_axis',(0.,-1.,0.));
#7144=DIRECTION('ref_axis',(0.,0.,-1.));
#7145=DIRECTION('',(0.,0.,-1.));
#7146=DIRECTION('',(1.,0.,0.));
#7147=DIRECTION('',(0.,0.,1.));
#7148=DIRECTION('center_axis',(0.,0.,1.));
#7149=DIRECTION('ref_axis',(0.,-1.,0.));
#7150=DIRECTION('',(0.,-1.,0.));
#7151=DIRECTION('',(1.,0.,0.));
#7152=DIRECTION('',(0.,1.,0.));
#7153=DIRECTION('center_axis',(0.,-1.,0.));
#7154=DIRECTION('ref_axis',(0.,0.,-1.));
#7155=DIRECTION('',(0.,0.,-1.));
#7156=DIRECTION('',(-1.,0.,0.));
#7157=DIRECTION('',(0.,0.,1.));
#7158=DIRECTION('center_axis',(1.,0.,0.));
#7159=DIRECTION('ref_axis',(0.,0.,-1.));
#7160=DIRECTION('',(1.,0.,0.));
#7161=DIRECTION('center_axis',(-1.,0.,0.));
#7162=DIRECTION('ref_axis',(0.,0.,-1.));
#7163=DIRECTION('center_axis',(0.,1.,0.));
#7164=DIRECTION('ref_axis',(0.,0.,1.));
#7165=DIRECTION('',(0.,0.,1.));
#7166=DIRECTION('',(1.,0.,0.));
#7167=DIRECTION('',(0.,0.,1.));
#7168=DIRECTION('center_axis',(0.,1.,0.));
#7169=DIRECTION('ref_axis',(0.,0.,1.));
#7170=DIRECTION('',(0.,0.,1.));
#7171=DIRECTION('',(1.,0.,0.));
#7172=DIRECTION('',(0.,0.,1.));
#7173=DIRECTION('center_axis',(0.,0.,-1.));
#7174=DIRECTION('ref_axis',(0.,1.,0.));
#7175=DIRECTION('',(0.,1.,0.));
#7176=DIRECTION('',(0.,1.,0.));
#7177=DIRECTION('center_axis',(0.,0.,-1.));
#7178=DIRECTION('ref_axis',(0.,1.,0.));
#7179=DIRECTION('',(0.,1.,0.));
#7180=DIRECTION('',(1.,0.,0.));
#7181=DIRECTION('',(0.,1.,0.));
#7182=DIRECTION('center_axis',(0.,-1.,0.));
#7183=DIRECTION('ref_axis',(0.,0.,-1.));
#7184=DIRECTION('',(0.,0.,-1.));
#7185=DIRECTION('',(0.,0.,-1.));
#7186=DIRECTION('center_axis',(0.,-1.,0.));
#7187=DIRECTION('ref_axis',(0.,0.,-1.));
#7188=DIRECTION('',(0.,0.,-1.));
#7189=DIRECTION('',(1.,0.,0.));
#7190=DIRECTION('',(0.,0.,-1.));
#7191=DIRECTION('center_axis',(0.,0.,1.));
#7192=DIRECTION('ref_axis',(0.,-1.,0.));
#7193=DIRECTION('',(0.,-1.,0.));
#7194=DIRECTION('',(0.,-1.,0.));
#7195=DIRECTION('center_axis',(0.,0.,1.));
#7196=DIRECTION('ref_axis',(0.,-1.,0.));
#7197=DIRECTION('',(0.,-1.,0.));
#7198=DIRECTION('',(0.,-1.,0.));
#7199=DIRECTION('center_axis',(1.,0.,0.));
#7200=DIRECTION('ref_axis',(0.,0.,-1.));
#7201=DIRECTION('center_axis',(1.,0.,0.));
#7202=DIRECTION('ref_axis',(0.,0.,-1.));
#8510=CARTESIAN_POINT('',(0.,0.,0.));
#8511=CARTESIAN_POINT('Origin',(4.,-1.1,0.));
#8512=CARTESIAN_POINT('',(3.725,-0.42,3.36777869765523E-17));
#8513=CARTESIAN_POINT('Origin',(4.,-0.42,0.));
#8514=CARTESIAN_POINT('',(3.725,-0.21,6.36764273396499E-17));
#8515=CARTESIAN_POINT('',(3.725,-1.1,3.36777869765523E-17));
#8516=CARTESIAN_POINT('',(3.82244719095435,-2.57175827820944E-17,0.21));
#8517=CARTESIAN_POINT('Ctrl Pts',(3.82244719095435,-3.81639164714898E-17,
0.21));
#8518=CARTESIAN_POINT('Ctrl Pts',(3.82244719095435,-0.0141630178371274,
0.21));
#8519=CARTESIAN_POINT('Ctrl Pts',(3.82070090566933,-0.0283388251429181,
0.208554382393535));
#8520=CARTESIAN_POINT('Ctrl Pts',(3.81433611385284,-0.0559106681449084,
0.202908887997328));
#8521=CARTESIAN_POINT('Ctrl Pts',(3.80974723471181,-0.0693141634661026,
0.198712082533353));
#8522=CARTESIAN_POINT('Ctrl Pts',(3.7937414503193,-0.107475484252795,0.182517999394844));
#8523=CARTESIAN_POINT('Ctrl Pts',(3.78023922617715,-0.130251970586776,0.166732877511574));
#8524=CARTESIAN_POINT('Ctrl Pts',(3.75710894103549,-0.166306329654162,0.130678518444188));
#8525=CARTESIAN_POINT('Ctrl Pts',(3.74560158587233,-0.182341144032027,0.107860332287474));
#8526=CARTESIAN_POINT('Ctrl Pts',(3.72949374752356,-0.204214038345313,0.0563806217319966));
#8527=CARTESIAN_POINT('Ctrl Pts',(3.725,-0.21,0.0276636393226111));
#8528=CARTESIAN_POINT('Ctrl Pts',(3.725,-0.21,0.));
#8529=CARTESIAN_POINT('',(3.725,0.21,9.8999995843689E-18));
#8530=CARTESIAN_POINT('Ctrl Pts',(3.725,0.21,-1.04083408558608E-17));
#8531=CARTESIAN_POINT('Ctrl Pts',(3.725,0.21,0.027663639322611));
#8532=CARTESIAN_POINT('Ctrl Pts',(3.72949374752356,0.204214038345313,0.0563806217319965));
#8533=CARTESIAN_POINT('Ctrl Pts',(3.74560158587233,0.182341144032027,0.107860332287474));
#8534=CARTESIAN_POINT('Ctrl Pts',(3.75710894103549,0.166306329654162,0.130678518444188));
#8535=CARTESIAN_POINT('Ctrl Pts',(3.78023922617715,0.130251970586776,0.166732877511574));
#8536=CARTESIAN_POINT('Ctrl Pts',(3.7937414503193,0.107475484252795,0.182517999394844));
#8537=CARTESIAN_POINT('Ctrl Pts',(3.80974723471181,0.0693141634661026,0.198712082533353));
#8538=CARTESIAN_POINT('Ctrl Pts',(3.81433611385284,0.0559106681449085,0.202908887997328));
#8539=CARTESIAN_POINT('Ctrl Pts',(3.82070090566933,0.0283388251429181,0.208554382393535));
#8540=CARTESIAN_POINT('Ctrl Pts',(3.82244719095435,0.0141630178371274,0.21));
#8541=CARTESIAN_POINT('Ctrl Pts',(3.82244719095435,3.46944695195361E-17,
0.21));
#8542=CARTESIAN_POINT('',(3.725,0.42,-3.36777869765523E-17));
#8543=CARTESIAN_POINT('',(3.725,-1.1,3.36777869765523E-17));
#8544=CARTESIAN_POINT('Origin',(4.,0.42,0.));
#8545=CARTESIAN_POINT('',(3.82244719095435,-3.46944695195361E-18,-0.21));
#8546=CARTESIAN_POINT('Ctrl Pts',(3.82244719095435,-3.46944695195361E-18,
-0.21));
#8547=CARTESIAN_POINT('Ctrl Pts',(3.82244719095435,0.0141630178371273,-0.21));
#8548=CARTESIAN_POINT('Ctrl Pts',(3.82070090566933,0.028338825142918,-0.208554382393535));
#8549=CARTESIAN_POINT('Ctrl Pts',(3.81433611385284,0.0559106681449083,-0.202908887997328));
#8550=CARTESIAN_POINT('Ctrl Pts',(3.80974723471181,0.0693141634661026,-0.198712082533353));
#8551=CARTESIAN_POINT('Ctrl Pts',(3.7937414503193,0.107475484252795,-0.182517999394844));
#8552=CARTESIAN_POINT('Ctrl Pts',(3.78023922617715,0.130251970586776,-0.166732877511574));
#8553=CARTESIAN_POINT('Ctrl Pts',(3.75710894103549,0.166306329654162,-0.130678518444188));
#8554=CARTESIAN_POINT('Ctrl Pts',(3.74560158587233,0.182341144032027,-0.107860332287474));
#8555=CARTESIAN_POINT('Ctrl Pts',(3.72949374752356,0.204214038345313,-0.0563806217319966));
#8556=CARTESIAN_POINT('Ctrl Pts',(3.725,0.21,-0.027663639322611));
#8557=CARTESIAN_POINT('Ctrl Pts',(3.725,0.21,2.77555756156289E-17));
#8558=CARTESIAN_POINT('Ctrl Pts',(3.725,-0.21,9.36750677027476E-17));
#8559=CARTESIAN_POINT('Ctrl Pts',(3.725,-0.21,-0.027663639322611));
#8560=CARTESIAN_POINT('Ctrl Pts',(3.72949374752356,-0.204214038345313,-0.0563806217319965));
#8561=CARTESIAN_POINT('Ctrl Pts',(3.74560158587233,-0.182341144032027,-0.107860332287474));
#8562=CARTESIAN_POINT('Ctrl Pts',(3.75710894103549,-0.166306329654162,-0.130678518444188));
#8563=CARTESIAN_POINT('Ctrl Pts',(3.78023922617715,-0.130251970586776,-0.166732877511574));
#8564=CARTESIAN_POINT('Ctrl Pts',(3.7937414503193,-0.107475484252795,-0.182517999394844));
#8565=CARTESIAN_POINT('Ctrl Pts',(3.80974723471181,-0.0693141634661024,
-0.198712082533353));
#8566=CARTESIAN_POINT('Ctrl Pts',(3.81433611385284,-0.0559106681449084,
-0.202908887997328));
#8567=CARTESIAN_POINT('Ctrl Pts',(3.82070090566933,-0.0283388251429182,
-0.208554382393535));
#8568=CARTESIAN_POINT('Ctrl Pts',(3.82244719095435,-0.0141630178371273,
-0.21));
#8569=CARTESIAN_POINT('Ctrl Pts',(3.82244719095435,-3.46944695195361E-18,
-0.21));
#8570=CARTESIAN_POINT('',(4.17755280904565,-3.12250225675825E-17,-0.21));
#8571=CARTESIAN_POINT('',(4.17755280904565,-2.57175827820944E-17,0.21));
#8572=CARTESIAN_POINT('Ctrl Pts',(4.17755280904565,-3.12250225675825E-17,
-0.21));
#8573=CARTESIAN_POINT('Ctrl Pts',(4.17755280904565,-0.0141630178371274,
-0.21));
#8574=CARTESIAN_POINT('Ctrl Pts',(4.17929909433067,-0.0283388251429182,
-0.208554382393535));
#8575=CARTESIAN_POINT('Ctrl Pts',(4.18566388614715,-0.0559106681449083,
-0.202908887997328));
#8576=CARTESIAN_POINT('Ctrl Pts',(4.19025276528819,-0.0693141634661022,
-0.198712082533353));
#8577=CARTESIAN_POINT('Ctrl Pts',(4.2062585496807,-0.107475484252795,-0.182517999394844));
#8578=CARTESIAN_POINT('Ctrl Pts',(4.21976077382285,-0.130251970586776,-0.166732877511574));
#8579=CARTESIAN_POINT('Ctrl Pts',(4.24289105896451,-0.166306329654162,-0.130678518444188));
#8580=CARTESIAN_POINT('Ctrl Pts',(4.25439841412767,-0.182341144032028,-0.107860332287473));
#8581=CARTESIAN_POINT('Ctrl Pts',(4.27050625247645,-0.204214038345313,-0.0563806217319961));
#8582=CARTESIAN_POINT('Ctrl Pts',(4.275,-0.21,-0.027663639322611));
#8583=CARTESIAN_POINT('Ctrl Pts',(4.275,-0.21,0.0276636393226111));
#8584=CARTESIAN_POINT('Ctrl Pts',(4.27050625247645,-0.204214038345313,0.0563806217319962));
#8585=CARTESIAN_POINT('Ctrl Pts',(4.25439841412767,-0.182341144032028,0.107860332287473));
#8586=CARTESIAN_POINT('Ctrl Pts',(4.24289105896451,-0.166306329654162,0.130678518444188));
#8587=CARTESIAN_POINT('Ctrl Pts',(4.21976077382285,-0.130251970586776,0.166732877511574));
#8588=CARTESIAN_POINT('Ctrl Pts',(4.2062585496807,-0.107475484252794,0.182517999394844));
#8589=CARTESIAN_POINT('Ctrl Pts',(4.19025276528819,-0.0693141634661021,
0.198712082533353));
#8590=CARTESIAN_POINT('Ctrl Pts',(4.18566388614715,-0.0559106681449083,
0.202908887997328));
#8591=CARTESIAN_POINT('Ctrl Pts',(4.17929909433067,-0.0283388251429182,
0.208554382393535));
#8592=CARTESIAN_POINT('Ctrl Pts',(4.17755280904565,-0.0141630178371274,
0.21));
#8593=CARTESIAN_POINT('Ctrl Pts',(4.17755280904565,-1.04083408558608E-17,
0.21));
#8594=CARTESIAN_POINT('Ctrl Pts',(4.17755280904565,1.38777878078145E-17,
0.21));
#8595=CARTESIAN_POINT('Ctrl Pts',(4.17755280904565,0.0141630178371274,0.21));
#8596=CARTESIAN_POINT('Ctrl Pts',(4.17929909433067,0.0283388251429182,0.208554382393535));
#8597=CARTESIAN_POINT('Ctrl Pts',(4.18566388614715,0.0559106681449083,0.202908887997328));
#8598=CARTESIAN_POINT('Ctrl Pts',(4.19025276528819,0.0693141634661021,0.198712082533353));
#8599=CARTESIAN_POINT('Ctrl Pts',(4.2062585496807,0.107475484252794,0.182517999394844));
#8600=CARTESIAN_POINT('Ctrl Pts',(4.21976077382285,0.130251970586776,0.166732877511574));
#8601=CARTESIAN_POINT('Ctrl Pts',(4.24289105896451,0.166306329654162,0.130678518444188));
#8602=CARTESIAN_POINT('Ctrl Pts',(4.25439841412767,0.182341144032028,0.107860332287473));
#8603=CARTESIAN_POINT('Ctrl Pts',(4.27050625247645,0.204214038345313,0.0563806217319961));
#8604=CARTESIAN_POINT('Ctrl Pts',(4.275,0.21,0.027663639322611));
#8605=CARTESIAN_POINT('Ctrl Pts',(4.275,0.21,-0.027663639322611));
#8606=CARTESIAN_POINT('Ctrl Pts',(4.27050625247645,0.204214038345313,-0.0563806217319961));
#8607=CARTESIAN_POINT('Ctrl Pts',(4.25439841412767,0.182341144032028,-0.107860332287473));
#8608=CARTESIAN_POINT('Ctrl Pts',(4.24289105896451,0.166306329654162,-0.130678518444188));
#8609=CARTESIAN_POINT('Ctrl Pts',(4.21976077382285,0.130251970586776,-0.166732877511574));
#8610=CARTESIAN_POINT('Ctrl Pts',(4.2062585496807,0.107475484252794,-0.182517999394844));
#8611=CARTESIAN_POINT('Ctrl Pts',(4.19025276528819,0.0693141634661021,-0.198712082533353));
#8612=CARTESIAN_POINT('Ctrl Pts',(4.18566388614715,0.0559106681449083,-0.202908887997328));
#8613=CARTESIAN_POINT('Ctrl Pts',(4.17929909433067,0.0283388251429182,-0.208554382393535));
#8614=CARTESIAN_POINT('Ctrl Pts',(4.17755280904565,0.0141630178371273,-0.21));
#8615=CARTESIAN_POINT('Ctrl Pts',(4.17755280904565,0.,-0.21));
#8616=CARTESIAN_POINT('Origin',(34.,-1.1,0.));
#8617=CARTESIAN_POINT('',(33.725,-0.42,3.3677786976552E-17));
#8618=CARTESIAN_POINT('Origin',(34.,-0.42,0.));
#8619=CARTESIAN_POINT('',(33.725,-0.21,4.28597456279281E-17));
#8620=CARTESIAN_POINT('',(33.725,-1.1,3.3677786976552E-17));
#8621=CARTESIAN_POINT('',(33.8224471909544,-2.57175827820944E-17,0.21));
#8622=CARTESIAN_POINT('Ctrl Pts',(33.8224471909543,-3.40005801291454E-16,
0.21));
#8623=CARTESIAN_POINT('Ctrl Pts',(33.8224471909543,-0.0141630178371276,
0.21));
#8624=CARTESIAN_POINT('Ctrl Pts',(33.8207009056693,-0.0283388251429169,
0.208554382393535));
#8625=CARTESIAN_POINT('Ctrl Pts',(33.8143361138529,-0.0559106681449082,
0.202908887997328));
#8626=CARTESIAN_POINT('Ctrl Pts',(33.8097472347118,-0.0693141634661021,
0.198712082533353));
#8627=CARTESIAN_POINT('Ctrl Pts',(33.7937414503193,-0.107475484252794,0.182517999394844));
#8628=CARTESIAN_POINT('Ctrl Pts',(33.7802392261772,-0.130251970586776,0.166732877511574));
#8629=CARTESIAN_POINT('Ctrl Pts',(33.7571089410355,-0.166306329654162,0.130678518444188));
#8630=CARTESIAN_POINT('Ctrl Pts',(33.7456015858723,-0.182341144032027,0.107860332287474));
#8631=CARTESIAN_POINT('Ctrl Pts',(33.7294937475236,-0.204214038345313,0.0563806217319973));
#8632=CARTESIAN_POINT('Ctrl Pts',(33.725,-0.21,0.027663639322611));
#8633=CARTESIAN_POINT('Ctrl Pts',(33.725,-0.21,-2.63677968348475E-16));
#8634=CARTESIAN_POINT('',(33.725,0.21,6.02069803876962E-17));
#8635=CARTESIAN_POINT('Ctrl Pts',(33.725,0.21,9.0205620750794E-17));
#8636=CARTESIAN_POINT('Ctrl Pts',(33.725,0.21,0.0276636393226113));
#8637=CARTESIAN_POINT('Ctrl Pts',(33.7294937475236,0.204214038345313,0.0563806217319973));
#8638=CARTESIAN_POINT('Ctrl Pts',(33.7456015858723,0.182341144032027,0.107860332287474));
#8639=CARTESIAN_POINT('Ctrl Pts',(33.7571089410355,0.166306329654162,0.130678518444188));
#8640=CARTESIAN_POINT('Ctrl Pts',(33.7802392261772,0.130251970586776,0.166732877511574));
#8641=CARTESIAN_POINT('Ctrl Pts',(33.7937414503193,0.107475484252794,0.182517999394844));
#8642=CARTESIAN_POINT('Ctrl Pts',(33.8097472347118,0.0693141634661021,0.198712082533353));
#8643=CARTESIAN_POINT('Ctrl Pts',(33.8143361138529,0.0559106681449082,0.202908887997328));
#8644=CARTESIAN_POINT('Ctrl Pts',(33.8207009056693,0.0283388251429169,0.208554382393535));
#8645=CARTESIAN_POINT('Ctrl Pts',(33.8224471909543,0.0141630178371276,0.21));
#8646=CARTESIAN_POINT('Ctrl Pts',(33.8224471909543,3.36536354339501E-16,
0.21));
#8647=CARTESIAN_POINT('',(33.725,0.42,-3.3677786976552E-17));
#8648=CARTESIAN_POINT('',(33.725,-1.1,3.3677786976552E-17));
#8649=CARTESIAN_POINT('Origin',(34.,0.42,0.));
#8650=CARTESIAN_POINT('',(33.8224471909543,2.67147415300428E-16,-0.21));
#8651=CARTESIAN_POINT('Ctrl Pts',(33.8224471909543,2.67147415300428E-16,
-0.21));
#8652=CARTESIAN_POINT('Ctrl Pts',(33.8224471909543,0.0141630178371276,-0.21));
#8653=CARTESIAN_POINT('Ctrl Pts',(33.8207009056693,0.028338825142917,-0.208554382393535));
#8654=CARTESIAN_POINT('Ctrl Pts',(33.8143361138529,0.0559106681449084,-0.202908887997328));
#8655=CARTESIAN_POINT('Ctrl Pts',(33.8097472347118,0.0693141634661022,-0.198712082533353));
#8656=CARTESIAN_POINT('Ctrl Pts',(33.7937414503193,0.107475484252794,-0.182517999394844));
#8657=CARTESIAN_POINT('Ctrl Pts',(33.7802392261772,0.130251970586776,-0.166732877511574));
#8658=CARTESIAN_POINT('Ctrl Pts',(33.7571089410355,0.166306329654162,-0.130678518444188));
#8659=CARTESIAN_POINT('Ctrl Pts',(33.7456015858723,0.182341144032027,-0.107860332287474));
#8660=CARTESIAN_POINT('Ctrl Pts',(33.7294937475236,0.204214038345313,-0.0563806217319973));
#8661=CARTESIAN_POINT('Ctrl Pts',(33.725,0.21,-0.0276636393226112));
#8662=CARTESIAN_POINT('Ctrl Pts',(33.725,0.21,-5.20417042793042E-18));
#8663=CARTESIAN_POINT('Ctrl Pts',(33.725,-0.21,4.5102810375397E-17));
#8664=CARTESIAN_POINT('Ctrl Pts',(33.725,-0.21,-0.0276636393226112));
#8665=CARTESIAN_POINT('Ctrl Pts',(33.7294937475236,-0.204214038345313,-0.0563806217319972));
#8666=CARTESIAN_POINT('Ctrl Pts',(33.7456015858723,-0.182341144032027,-0.107860332287474));
#8667=CARTESIAN_POINT('Ctrl Pts',(33.7571089410355,-0.166306329654162,-0.130678518444188));
#8668=CARTESIAN_POINT('Ctrl Pts',(33.7802392261772,-0.130251970586776,-0.166732877511574));
#8669=CARTESIAN_POINT('Ctrl Pts',(33.7937414503193,-0.107475484252794,-0.182517999394844));
#8670=CARTESIAN_POINT('Ctrl Pts',(33.8097472347118,-0.0693141634661023,
-0.198712082533353));
#8671=CARTESIAN_POINT('Ctrl Pts',(33.8143361138529,-0.0559106681449084,
-0.202908887997328));
#8672=CARTESIAN_POINT('Ctrl Pts',(33.8207009056693,-0.028338825142917,-0.208554382393535));
#8673=CARTESIAN_POINT('Ctrl Pts',(33.8224471909544,-0.0141630178371271,
-0.21));
#8674=CARTESIAN_POINT('Ctrl Pts',(33.8224471909544,2.63677968348475E-16,
-0.21));
#8675=CARTESIAN_POINT('',(34.1775528090457,-1.94289029309402E-16,-0.21));
#8676=CARTESIAN_POINT('',(34.1775528090456,-2.57175827820944E-17,0.21));
#8677=CARTESIAN_POINT('Ctrl Pts',(34.1775528090457,-1.94289029309402E-16,
-0.21));
#8678=CARTESIAN_POINT('Ctrl Pts',(34.1775528090457,-0.0141630178371275,
-0.21));
#8679=CARTESIAN_POINT('Ctrl Pts',(34.1792990943307,-0.028338825142917,-0.208554382393535));
#8680=CARTESIAN_POINT('Ctrl Pts',(34.1856638861471,-0.0559106681449084,
-0.202908887997328));
#8681=CARTESIAN_POINT('Ctrl Pts',(34.1902527652882,-0.0693141634661023,
-0.198712082533353));
#8682=CARTESIAN_POINT('Ctrl Pts',(34.2062585496807,-0.107475484252794,-0.182517999394844));
#8683=CARTESIAN_POINT('Ctrl Pts',(34.2197607738228,-0.130251970586776,-0.166732877511574));
#8684=CARTESIAN_POINT('Ctrl Pts',(34.2428910589645,-0.166306329654162,-0.130678518444188));
#8685=CARTESIAN_POINT('Ctrl Pts',(34.2543984141277,-0.182341144032027,-0.107860332287474));
#8686=CARTESIAN_POINT('Ctrl Pts',(34.2705062524764,-0.204214038345313,-0.0563806217319973));
#8687=CARTESIAN_POINT('Ctrl Pts',(34.275,-0.21,-0.0276636393226112));
#8688=CARTESIAN_POINT('Ctrl Pts',(34.275,-0.21,0.0276636393226113));
#8689=CARTESIAN_POINT('Ctrl Pts',(34.2705062524764,-0.204214038345313,0.0563806217319974));
#8690=CARTESIAN_POINT('Ctrl Pts',(34.2543984141277,-0.182341144032027,0.107860332287474));
#8691=CARTESIAN_POINT('Ctrl Pts',(34.2428910589645,-0.166306329654162,0.130678518444188));
#8692=CARTESIAN_POINT('Ctrl Pts',(34.2197607738228,-0.130251970586776,0.166732877511574));
#8693=CARTESIAN_POINT('Ctrl Pts',(34.2062585496807,-0.107475484252794,0.182517999394844));
#8694=CARTESIAN_POINT('Ctrl Pts',(34.1902527652882,-0.0693141634661023,
0.198712082533353));
#8695=CARTESIAN_POINT('Ctrl Pts',(34.1856638861471,-0.0559106681449084,
0.202908887997328));
#8696=CARTESIAN_POINT('Ctrl Pts',(34.1792990943307,-0.028338825142917,0.208554382393535));
#8697=CARTESIAN_POINT('Ctrl Pts',(34.1775528090457,-0.0141630178371273,
0.21));
#8698=CARTESIAN_POINT('Ctrl Pts',(34.1775528090457,1.04083408558608E-17,
0.21));
#8699=CARTESIAN_POINT('Ctrl Pts',(34.1775528090457,-1.38777878078145E-17,
0.21));
#8700=CARTESIAN_POINT('Ctrl Pts',(34.1775528090457,0.0141630178371273,0.21));
#8701=CARTESIAN_POINT('Ctrl Pts',(34.1792990943307,0.028338825142917,0.208554382393535));
#8702=CARTESIAN_POINT('Ctrl Pts',(34.1856638861471,0.0559106681449084,0.202908887997328));
#8703=CARTESIAN_POINT('Ctrl Pts',(34.1902527652882,0.0693141634661023,0.198712082533353));
#8704=CARTESIAN_POINT('Ctrl Pts',(34.2062585496807,0.107475484252794,0.182517999394844));
#8705=CARTESIAN_POINT('Ctrl Pts',(34.2197607738228,0.130251970586776,0.166732877511574));
#8706=CARTESIAN_POINT('Ctrl Pts',(34.2428910589645,0.166306329654162,0.130678518444188));
#8707=CARTESIAN_POINT('Ctrl Pts',(34.2543984141277,0.182341144032027,0.107860332287474));
#8708=CARTESIAN_POINT('Ctrl Pts',(34.2705062524764,0.204214038345313,0.0563806217319973));
#8709=CARTESIAN_POINT('Ctrl Pts',(34.275,0.21,0.0276636393226112));
#8710=CARTESIAN_POINT('Ctrl Pts',(34.275,0.21,-0.0276636393226112));
#8711=CARTESIAN_POINT('Ctrl Pts',(34.2705062524764,0.204214038345313,-0.0563806217319973));
#8712=CARTESIAN_POINT('Ctrl Pts',(34.2543984141277,0.182341144032027,-0.107860332287474));
#8713=CARTESIAN_POINT('Ctrl Pts',(34.2428910589645,0.166306329654162,-0.130678518444188));
#8714=CARTESIAN_POINT('Ctrl Pts',(34.2197607738228,0.130251970586776,-0.166732877511574));
#8715=CARTESIAN_POINT('Ctrl Pts',(34.2062585496807,0.107475484252794,-0.182517999394844));
#8716=CARTESIAN_POINT('Ctrl Pts',(34.1902527652882,0.0693141634661022,-0.198712082533353));
#8717=CARTESIAN_POINT('Ctrl Pts',(34.1856638861471,0.0559106681449084,-0.202908887997328));
#8718=CARTESIAN_POINT('Ctrl Pts',(34.1792990943307,0.028338825142917,-0.208554382393535));
#8719=CARTESIAN_POINT('Ctrl Pts',(34.1775528090456,0.0141630178371274,-0.21));
#8720=CARTESIAN_POINT('Ctrl Pts',(34.1775528090456,1.00613961606655E-16,
-0.21));
#8721=CARTESIAN_POINT('Origin',(-0.1,0.,0.));
#8722=CARTESIAN_POINT('',(-0.1,-2.57175827820944E-17,0.21));
#8723=CARTESIAN_POINT('Origin',(-0.1,0.,0.));
#8724=CARTESIAN_POINT('',(1.17755280904565,0.21,-3.46944695195361E-18));
#8725=CARTESIAN_POINT('',(1.275,-2.45045053518637E-18,0.21));
#8726=CARTESIAN_POINT('Ctrl Pts',(1.17755280904565,0.21,-3.46944695195361E-18));
#8727=CARTESIAN_POINT('Ctrl Pts',(1.17755280904565,0.21,-0.0141630178371274));
#8728=CARTESIAN_POINT('Ctrl Pts',(1.17929909433067,0.208554382393535,-0.0283388251429181));
#8729=CARTESIAN_POINT('Ctrl Pts',(1.18566388614715,0.202908887997328,-0.0559106681449085));
#8730=CARTESIAN_POINT('Ctrl Pts',(1.19025276528819,0.198712082533353,-0.0693141634661026));
#8731=CARTESIAN_POINT('Ctrl Pts',(1.2062585496807,0.182517999394844,-0.107475484252795));
#8732=CARTESIAN_POINT('Ctrl Pts',(1.21976077382285,0.166732877511574,-0.130251970586776));
#8733=CARTESIAN_POINT('Ctrl Pts',(1.24289105896451,0.130678518444188,-0.166306329654162));
#8734=CARTESIAN_POINT('Ctrl Pts',(1.25439841412767,0.107860332287473,-0.182341144032028));
#8735=CARTESIAN_POINT('Ctrl Pts',(1.27050625247644,0.0563806217319963,-0.204214038345313));
#8736=CARTESIAN_POINT('Ctrl Pts',(1.275,0.027663639322611,-0.21));
#8737=CARTESIAN_POINT('Ctrl Pts',(1.275,-0.0276636393226111,-0.21));
#8738=CARTESIAN_POINT('Ctrl Pts',(1.27050625247644,-0.0563806217319964,
-0.204214038345313));
#8739=CARTESIAN_POINT('Ctrl Pts',(1.25439841412767,-0.107860332287474,-0.182341144032027));
#8740=CARTESIAN_POINT('Ctrl Pts',(1.24289105896451,-0.130678518444188,-0.166306329654162));
#8741=CARTESIAN_POINT('Ctrl Pts',(1.21976077382284,-0.166732877511574,-0.130251970586776));
#8742=CARTESIAN_POINT('Ctrl Pts',(1.2062585496807,-0.182517999394844,-0.107475484252795));
#8743=CARTESIAN_POINT('Ctrl Pts',(1.19025276528819,-0.198712082533353,-0.0693141634661024));
#8744=CARTESIAN_POINT('Ctrl Pts',(1.18566388614715,-0.202908887997328,-0.0559106681449083));
#8745=CARTESIAN_POINT('Ctrl Pts',(1.17929909433067,-0.208554382393535,-0.0283388251429181));
#8746=CARTESIAN_POINT('Ctrl Pts',(1.17755280904565,-0.21,-0.0141630178371274));
#8747=CARTESIAN_POINT('Ctrl Pts',(1.17755280904565,-0.21,0.0141630178371274));
#8748=CARTESIAN_POINT('Ctrl Pts',(1.17929909433067,-0.208554382393535,0.0283388251429181));
#8749=CARTESIAN_POINT('Ctrl Pts',(1.18566388614715,-0.202908887997328,0.0559106681449083));
#8750=CARTESIAN_POINT('Ctrl Pts',(1.19025276528819,-0.198712082533353,0.0693141634661024));
#8751=CARTESIAN_POINT('Ctrl Pts',(1.2062585496807,-0.182517999394844,0.107475484252795));
#8752=CARTESIAN_POINT('Ctrl Pts',(1.21976077382284,-0.166732877511574,0.130251970586776));
#8753=CARTESIAN_POINT('Ctrl Pts',(1.24289105896451,-0.130678518444188,0.166306329654162));
#8754=CARTESIAN_POINT('Ctrl Pts',(1.25439841412767,-0.107860332287473,0.182341144032027));
#8755=CARTESIAN_POINT('Ctrl Pts',(1.27050625247644,-0.0563806217319963,
0.204214038345313));
#8756=CARTESIAN_POINT('Ctrl Pts',(1.275,-0.027663639322611,0.21));
#8757=CARTESIAN_POINT('Ctrl Pts',(1.275,4.16333634234434E-17,0.21));
#8758=CARTESIAN_POINT('',(-0.1,-2.57175827820944E-17,0.21));
#8759=CARTESIAN_POINT('Ctrl Pts',(1.275,2.77555756156289E-17,0.21));
#8760=CARTESIAN_POINT('Ctrl Pts',(1.275,0.0276636393226111,0.21));
#8761=CARTESIAN_POINT('Ctrl Pts',(1.27050625247644,0.0563806217319964,0.204214038345313));
#8762=CARTESIAN_POINT('Ctrl Pts',(1.25439841412767,0.107860332287474,0.182341144032027));
#8763=CARTESIAN_POINT('Ctrl Pts',(1.24289105896451,0.130678518444188,0.166306329654162));
#8764=CARTESIAN_POINT('Ctrl Pts',(1.21976077382284,0.166732877511574,0.130251970586776));
#8765=CARTESIAN_POINT('Ctrl Pts',(1.2062585496807,0.182517999394844,0.107475484252795));
#8766=CARTESIAN_POINT('Ctrl Pts',(1.19025276528819,0.198712082533353,0.0693141634661023));
#8767=CARTESIAN_POINT('Ctrl Pts',(1.18566388614715,0.202908887997328,0.0559106681449083));
#8768=CARTESIAN_POINT('Ctrl Pts',(1.17929909433067,0.208554382393535,0.0283388251429181));
#8769=CARTESIAN_POINT('Ctrl Pts',(1.17755280904565,0.21,0.0141630178371273));
#8770=CARTESIAN_POINT('Ctrl Pts',(1.17755280904565,0.21,-1.38777878078145E-17));
#8771=CARTESIAN_POINT('Origin',(1.,0.,-1.1));
#8772=CARTESIAN_POINT('',(0.725,-3.36777869765522E-17,-0.42));
#8773=CARTESIAN_POINT('Origin',(1.,0.,-0.42));
#8774=CARTESIAN_POINT('',(0.725,-3.76555751999978E-17,-0.21));
#8775=CARTESIAN_POINT('',(0.725,-3.36777869765522E-17,-1.1));
#8776=CARTESIAN_POINT('',(0.725,-6.43055263241525E-18,0.21));
#8777=CARTESIAN_POINT('Ctrl Pts',(0.725,2.08166817117217E-17,0.21));
#8778=CARTESIAN_POINT('Ctrl Pts',(0.725,-0.027663639322611,0.21));
#8779=CARTESIAN_POINT('Ctrl Pts',(0.729493747523555,-0.0563806217319963,
0.204214038345313));
#8780=CARTESIAN_POINT('Ctrl Pts',(0.74560158587233,-0.107860332287473,0.182341144032027));
#8781=CARTESIAN_POINT('Ctrl Pts',(0.757108941035492,-0.130678518444188,
0.166306329654162));
#8782=CARTESIAN_POINT('Ctrl Pts',(0.780239226177155,-0.166732877511574,
0.130251970586776));
#8783=CARTESIAN_POINT('Ctrl Pts',(0.793741450319299,-0.182517999394844,
0.107475484252795));
#8784=CARTESIAN_POINT('Ctrl Pts',(0.809747234711808,-0.198712082533353,
0.0693141634661026));
#8785=CARTESIAN_POINT('Ctrl Pts',(0.814336113852846,-0.202908887997328,
0.0559106681449084));
#8786=CARTESIAN_POINT('Ctrl Pts',(0.820700905669331,-0.208554382393535,
0.028338825142918));
#8787=CARTESIAN_POINT('Ctrl Pts',(0.822447190954353,-0.21,0.0141630178371274));
#8788=CARTESIAN_POINT('Ctrl Pts',(0.822447190954353,-0.21,-0.0141630178371273));
#8789=CARTESIAN_POINT('Ctrl Pts',(0.820700905669331,-0.208554382393535,
-0.028338825142918));
#8790=CARTESIAN_POINT('Ctrl Pts',(0.814336113852846,-0.202908887997328,
-0.0559106681449083));
#8791=CARTESIAN_POINT('Ctrl Pts',(0.809747234711808,-0.198712082533353,
-0.0693141634661024));
#8792=CARTESIAN_POINT('Ctrl Pts',(0.7937414503193,-0.182517999394844,-0.107475484252795));
#8793=CARTESIAN_POINT('Ctrl Pts',(0.780239226177155,-0.166732877511574,
-0.130251970586776));
#8794=CARTESIAN_POINT('Ctrl Pts',(0.757108941035492,-0.130678518444188,
-0.166306329654162));
#8795=CARTESIAN_POINT('Ctrl Pts',(0.74560158587233,-0.107860332287474,-0.182341144032027));
#8796=CARTESIAN_POINT('Ctrl Pts',(0.729493747523555,-0.0563806217319965,
-0.204214038345313));
#8797=CARTESIAN_POINT('Ctrl Pts',(0.725,-0.0276636393226112,-0.21));
#8798=CARTESIAN_POINT('Ctrl Pts',(0.725,-9.71445146547012E-17,-0.21));
#8799=CARTESIAN_POINT('',(0.725,3.36777869765522E-17,0.42));
#8800=CARTESIAN_POINT('',(0.725,-3.36777869765522E-17,-1.1));
#8801=CARTESIAN_POINT('Origin',(1.,0.,0.42));
#8802=CARTESIAN_POINT('',(0.822447190954353,0.21,0.));
#8803=CARTESIAN_POINT('Ctrl Pts',(0.822447190954353,0.21,0.));
#8804=CARTESIAN_POINT('Ctrl Pts',(0.822447190954353,0.21,0.0141630178371274));
#8805=CARTESIAN_POINT('Ctrl Pts',(0.820700905669331,0.208554382393535,0.0283388251429181));
#8806=CARTESIAN_POINT('Ctrl Pts',(0.814336113852846,0.202908887997328,0.0559106681449084));
#8807=CARTESIAN_POINT('Ctrl Pts',(0.809747234711808,0.198712082533353,0.0693141634661024));
#8808=CARTESIAN_POINT('Ctrl Pts',(0.793741450319299,0.182517999394844,0.107475484252795));
#8809=CARTESIAN_POINT('Ctrl Pts',(0.780239226177155,0.166732877511574,0.130251970586776));
#8810=CARTESIAN_POINT('Ctrl Pts',(0.757108941035492,0.130678518444188,0.166306329654162));
#8811=CARTESIAN_POINT('Ctrl Pts',(0.74560158587233,0.107860332287474,0.182341144032027));
#8812=CARTESIAN_POINT('Ctrl Pts',(0.729493747523555,0.0563806217319964,
0.204214038345313));
#8813=CARTESIAN_POINT('Ctrl Pts',(0.725,0.0276636393226111,0.21));
#8814=CARTESIAN_POINT('Ctrl Pts',(0.725,2.77555756156289E-17,0.21));
#8815=CARTESIAN_POINT('Ctrl Pts',(0.725,-4.16333634234434E-17,-0.21));
#8816=CARTESIAN_POINT('Ctrl Pts',(0.725,0.027663639322611,-0.21));
#8817=CARTESIAN_POINT('Ctrl Pts',(0.729493747523555,0.0563806217319963,
-0.204214038345313));
#8818=CARTESIAN_POINT('Ctrl Pts',(0.74560158587233,0.107860332287473,-0.182341144032028));
#8819=CARTESIAN_POINT('Ctrl Pts',(0.757108941035492,0.130678518444188,-0.166306329654162));
#8820=CARTESIAN_POINT('Ctrl Pts',(0.780239226177155,0.166732877511574,-0.130251970586776));
#8821=CARTESIAN_POINT('Ctrl Pts',(0.793741450319299,0.182517999394844,-0.107475484252795));
#8822=CARTESIAN_POINT('Ctrl Pts',(0.809747234711808,0.198712082533353,-0.0693141634661025));
#8823=CARTESIAN_POINT('Ctrl Pts',(0.814336113852846,0.202908887997328,-0.0559106681449083));
#8824=CARTESIAN_POINT('Ctrl Pts',(0.820700905669331,0.208554382393535,-0.0283388251429181));
#8825=CARTESIAN_POINT('Ctrl Pts',(0.822447190954353,0.21,-0.0141630178371273));
#8826=CARTESIAN_POINT('Ctrl Pts',(0.822447190954353,0.21,6.93889390390723E-18));
#8827=CARTESIAN_POINT('Origin',(37.,0.,-1.1));
#8828=CARTESIAN_POINT('',(36.725,-3.3677786976552E-17,-0.42));
#8829=CARTESIAN_POINT('Origin',(37.,0.,-0.42));
#8830=CARTESIAN_POINT('',(36.725,2.05205711436755E-16,-0.21));
#8831=CARTESIAN_POINT('',(36.725,-3.3677786976552E-17,-1.1));
#8832=CARTESIAN_POINT('',(36.725,-7.0615321243557E-17,0.21));
#8833=CARTESIAN_POINT('Ctrl Pts',(36.725,-9.71445146547012E-17,0.21));
#8834=CARTESIAN_POINT('Ctrl Pts',(36.725,-0.0276636393226113,0.21));
#8835=CARTESIAN_POINT('Ctrl Pts',(36.7294937475236,-0.0563806217319973,
0.204214038345313));
#8836=CARTESIAN_POINT('Ctrl Pts',(36.7456015858723,-0.107860332287474,0.182341144032027));
#8837=CARTESIAN_POINT('Ctrl Pts',(36.7571089410355,-0.130678518444188,0.166306329654162));
#8838=CARTESIAN_POINT('Ctrl Pts',(36.7802392261772,-0.166732877511574,0.130251970586776));
#8839=CARTESIAN_POINT('Ctrl Pts',(36.7937414503193,-0.182517999394844,0.107475484252794));
#8840=CARTESIAN_POINT('Ctrl Pts',(36.8097472347118,-0.198712082533353,0.0693141634661021));
#8841=CARTESIAN_POINT('Ctrl Pts',(36.8143361138529,-0.202908887997328,0.0559106681449082));
#8842=CARTESIAN_POINT('Ctrl Pts',(36.8207009056693,-0.208554382393535,0.0283388251429169));
#8843=CARTESIAN_POINT('Ctrl Pts',(36.8224471909544,-0.21,0.0141630178371273));
#8844=CARTESIAN_POINT('Ctrl Pts',(36.8224471909544,-0.21,-0.0141630178371273));
#8845=CARTESIAN_POINT('Ctrl Pts',(36.8207009056693,-0.208554382393535,-0.0283388251429169));
#8846=CARTESIAN_POINT('Ctrl Pts',(36.8143361138529,-0.202908887997328,-0.0559106681449082));
#8847=CARTESIAN_POINT('Ctrl Pts',(36.8097472347118,-0.198712082533353,-0.0693141634661022));
#8848=CARTESIAN_POINT('Ctrl Pts',(36.7937414503193,-0.182517999394844,-0.107475484252794));
#8849=CARTESIAN_POINT('Ctrl Pts',(36.7802392261772,-0.166732877511574,-0.130251970586776));
#8850=CARTESIAN_POINT('Ctrl Pts',(36.7571089410355,-0.130678518444188,-0.166306329654162));
#8851=CARTESIAN_POINT('Ctrl Pts',(36.7456015858723,-0.107860332287474,-0.182341144032027));
#8852=CARTESIAN_POINT('Ctrl Pts',(36.7294937475236,-0.0563806217319974,
-0.204214038345313));
#8853=CARTESIAN_POINT('Ctrl Pts',(36.725,-0.0276636393226115,-0.21));
#8854=CARTESIAN_POINT('Ctrl Pts',(36.725,-2.84494650060196E-16,-0.21));
#8855=CARTESIAN_POINT('',(36.725,3.3677786976552E-17,0.42));
#8856=CARTESIAN_POINT('',(36.725,-3.3677786976552E-17,-1.1));
#8857=CARTESIAN_POINT('Origin',(37.,0.,0.42));
#8858=CARTESIAN_POINT('',(36.8224471909543,0.21,1.49186218934005E-16));
#8859=CARTESIAN_POINT('Ctrl Pts',(36.8224471909543,0.21,1.49186218934005E-16));
#8860=CARTESIAN_POINT('Ctrl Pts',(36.8224471909543,0.21,0.0141630178371275));
#8861=CARTESIAN_POINT('Ctrl Pts',(36.8207009056693,0.208554382393535,0.028338825142917));
#8862=CARTESIAN_POINT('Ctrl Pts',(36.8143361138529,0.202908887997328,0.0559106681449084));
#8863=CARTESIAN_POINT('Ctrl Pts',(36.8097472347118,0.198712082533353,0.0693141634661022));
#8864=CARTESIAN_POINT('Ctrl Pts',(36.7937414503193,0.182517999394844,0.107475484252794));
#8865=CARTESIAN_POINT('Ctrl Pts',(36.7802392261772,0.166732877511574,0.130251970586776));
#8866=CARTESIAN_POINT('Ctrl Pts',(36.7571089410355,0.130678518444188,0.166306329654162));
#8867=CARTESIAN_POINT('Ctrl Pts',(36.7456015858723,0.107860332287474,0.182341144032027));
#8868=CARTESIAN_POINT('Ctrl Pts',(36.7294937475236,0.0563806217319973,0.204214038345313));
#8869=CARTESIAN_POINT('Ctrl Pts',(36.725,0.0276636393226112,0.21));
#8870=CARTESIAN_POINT('Ctrl Pts',(36.725,2.08166817117217E-17,0.21));
#8871=CARTESIAN_POINT('Ctrl Pts',(36.725,2.08166817117217E-16,-0.21));
#8872=CARTESIAN_POINT('Ctrl Pts',(36.725,0.0276636393226114,-0.21));
#8873=CARTESIAN_POINT('Ctrl Pts',(36.7294937475236,0.0563806217319972,-0.204214038345313));
#8874=CARTESIAN_POINT('Ctrl Pts',(36.7456015858723,0.107860332287474,-0.182341144032027));
#8875=CARTESIAN_POINT('Ctrl Pts',(36.7571089410355,0.130678518444188,-0.166306329654162));
#8876=CARTESIAN_POINT('Ctrl Pts',(36.7802392261772,0.166732877511574,-0.130251970586776));
#8877=CARTESIAN_POINT('Ctrl Pts',(36.7937414503193,0.182517999394844,-0.107475484252794));
#8878=CARTESIAN_POINT('Ctrl Pts',(36.8097472347118,0.198712082533353,-0.0693141634661023));
#8879=CARTESIAN_POINT('Ctrl Pts',(36.8143361138529,0.202908887997328,-0.0559106681449084));
#8880=CARTESIAN_POINT('Ctrl Pts',(36.8207009056693,0.208554382393535,-0.028338825142917));
#8881=CARTESIAN_POINT('Ctrl Pts',(36.8224471909543,0.21,-0.0141630178371273));
#8882=CARTESIAN_POINT('Ctrl Pts',(36.8224471909543,0.21,5.55111512312578E-17));
#8883=CARTESIAN_POINT('',(37.1775528090456,0.21,-1.73472347597681E-18));
#8884=CARTESIAN_POINT('',(37.275,-4.32661872577435E-16,0.21));
#8885=CARTESIAN_POINT('Ctrl Pts',(37.1775528090456,0.21,-1.73472347597681E-18));
#8886=CARTESIAN_POINT('Ctrl Pts',(37.1775528090456,0.21,-0.0141630178371273));
#8887=CARTESIAN_POINT('Ctrl Pts',(37.1792990943307,0.208554382393535,-0.028338825142917));
#8888=CARTESIAN_POINT('Ctrl Pts',(37.1856638861471,0.202908887997328,-0.0559106681449084));
#8889=CARTESIAN_POINT('Ctrl Pts',(37.1902527652882,0.198712082533353,-0.0693141634661023));
#8890=CARTESIAN_POINT('Ctrl Pts',(37.2062585496807,0.182517999394844,-0.107475484252794));
#8891=CARTESIAN_POINT('Ctrl Pts',(37.2197607738228,0.166732877511574,-0.130251970586776));
#8892=CARTESIAN_POINT('Ctrl Pts',(37.2428910589645,0.130678518444188,-0.166306329654162));
#8893=CARTESIAN_POINT('Ctrl Pts',(37.2543984141277,0.107860332287474,-0.182341144032027));
#8894=CARTESIAN_POINT('Ctrl Pts',(37.2705062524764,0.0563806217319972,-0.204214038345313));
#8895=CARTESIAN_POINT('Ctrl Pts',(37.275,0.0276636393226112,-0.21));
#8896=CARTESIAN_POINT('Ctrl Pts',(37.275,-0.0276636393226113,-0.21));
#8897=CARTESIAN_POINT('Ctrl Pts',(37.2705062524764,-0.0563806217319974,
-0.204214038345313));
#8898=CARTESIAN_POINT('Ctrl Pts',(37.2543984141277,-0.107860332287474,-0.182341144032027));
#8899=CARTESIAN_POINT('Ctrl Pts',(37.2428910589645,-0.130678518444188,-0.166306329654162));
#8900=CARTESIAN_POINT('Ctrl Pts',(37.2197607738228,-0.166732877511574,-0.130251970586776));
#8901=CARTESIAN_POINT('Ctrl Pts',(37.2062585496807,-0.182517999394844,-0.107475484252794));
#8902=CARTESIAN_POINT('Ctrl Pts',(37.1902527652882,-0.198712082533353,-0.0693141634661022));
#8903=CARTESIAN_POINT('Ctrl Pts',(37.1856638861471,-0.202908887997328,-0.0559106681449083));
#8904=CARTESIAN_POINT('Ctrl Pts',(37.1792990943307,-0.208554382393535,-0.028338825142917));
#8905=CARTESIAN_POINT('Ctrl Pts',(37.1775528090456,-0.21,-0.0141630178371273));
#8906=CARTESIAN_POINT('Ctrl Pts',(37.1775528090456,-0.21,0.0141630178371273));
#8907=CARTESIAN_POINT('Ctrl Pts',(37.1792990943307,-0.208554382393535,0.028338825142917));
#8908=CARTESIAN_POINT('Ctrl Pts',(37.1856638861471,-0.202908887997328,0.0559106681449084));
#8909=CARTESIAN_POINT('Ctrl Pts',(37.1902527652882,-0.198712082533353,0.0693141634661023));
#8910=CARTESIAN_POINT('Ctrl Pts',(37.2062585496807,-0.182517999394844,0.107475484252794));
#8911=CARTESIAN_POINT('Ctrl Pts',(37.2197607738228,-0.166732877511574,0.130251970586776));
#8912=CARTESIAN_POINT('Ctrl Pts',(37.2428910589645,-0.130678518444188,0.166306329654162));
#8913=CARTESIAN_POINT('Ctrl Pts',(37.2543984141277,-0.107860332287474,0.182341144032027));
#8914=CARTESIAN_POINT('Ctrl Pts',(37.2705062524764,-0.0563806217319973,
0.204214038345313));
#8915=CARTESIAN_POINT('Ctrl Pts',(37.275,-0.0276636393226111,0.21));
#8916=CARTESIAN_POINT('Ctrl Pts',(37.275,1.04083408558608E-16,0.21));
#8917=CARTESIAN_POINT('Ctrl Pts',(37.275,-7.97972798949331E-17,0.21));
#8918=CARTESIAN_POINT('Ctrl Pts',(37.275,0.0276636393226111,0.21));
#8919=CARTESIAN_POINT('Ctrl Pts',(37.2705062524764,0.0563806217319973,0.204214038345313));
#8920=CARTESIAN_POINT('Ctrl Pts',(37.2543984141277,0.107860332287474,0.182341144032027));
#8921=CARTESIAN_POINT('Ctrl Pts',(37.2428910589645,0.130678518444188,0.166306329654162));
#8922=CARTESIAN_POINT('Ctrl Pts',(37.2197607738228,0.166732877511574,0.130251970586776));
#8923=CARTESIAN_POINT('Ctrl Pts',(37.2062585496807,0.182517999394844,0.107475484252794));
#8924=CARTESIAN_POINT('Ctrl Pts',(37.1902527652882,0.198712082533353,0.0693141634661022));
#8925=CARTESIAN_POINT('Ctrl Pts',(37.1856638861471,0.202908887997328,0.0559106681449083));
#8926=CARTESIAN_POINT('Ctrl Pts',(37.1792990943307,0.208554382393535,0.028338825142917));
#8927=CARTESIAN_POINT('Ctrl Pts',(37.1775528090457,0.21,0.0141630178371273));
#8928=CARTESIAN_POINT('Ctrl Pts',(37.1775528090457,0.21,-1.04083408558608E-17));
#8929=CARTESIAN_POINT('Origin',(-0.1,0.,0.));
#8930=CARTESIAN_POINT('',(-0.1,-2.57175827820944E-17,0.21));
#8931=CARTESIAN_POINT('Origin',(-0.1,0.,0.));
#8932=CARTESIAN_POINT('',(0.,-2.57175827820944E-17,0.21));
#8933=CARTESIAN_POINT('Origin',(0.,0.,0.));
#8934=CARTESIAN_POINT('',(-0.1,-2.57175827820944E-17,0.21));
#8935=CARTESIAN_POINT('Origin',(-0.1,0.82,-0.3));
#8936=CARTESIAN_POINT('',(0.,0.82,-0.3));
#8937=CARTESIAN_POINT('',(0.,1.,-0.3));
#8938=CARTESIAN_POINT('',(0.,0.41,-0.3));
#8939=CARTESIAN_POINT('',(40.,0.82,-0.3));
#8940=CARTESIAN_POINT('',(-0.1,0.82,-0.3));
#8941=CARTESIAN_POINT('',(40.,1.,-0.3));
#8942=CARTESIAN_POINT('',(40.,0.41,-0.3));
#8943=CARTESIAN_POINT('',(-0.05,1.,-0.3));
#8944=CARTESIAN_POINT('Origin',(-0.1,0.82,-0.55));
#8945=CARTESIAN_POINT('',(0.,0.82,-0.55));
#8946=CARTESIAN_POINT('',(0.,0.82,-0.275));
#8947=CARTESIAN_POINT('',(40.,0.82,-0.55));
#8948=CARTESIAN_POINT('',(-0.1,0.82,-0.55));
#8949=CARTESIAN_POINT('',(40.,0.82,-0.275));
#8950=CARTESIAN_POINT('Origin',(-0.1,0.67,-0.55));
#8951=CARTESIAN_POINT('',(0.,0.67,-0.55));
#8952=CARTESIAN_POINT('',(0.,0.335,-0.55));
#8953=CARTESIAN_POINT('',(40.,0.67,-0.55));
#8954=CARTESIAN_POINT('',(-0.1,0.67,-0.55));
#8955=CARTESIAN_POINT('',(40.,0.335,-0.55));
#8956=CARTESIAN_POINT('Origin',(-0.1,0.42,-0.3));
#8957=CARTESIAN_POINT('',(0.,0.42,-0.3));
#8958=CARTESIAN_POINT('',(0.,0.24,-0.12));
#8959=CARTESIAN_POINT('',(40.,0.42,-0.3));
#8960=CARTESIAN_POINT('',(-0.1,0.42,-0.3));
#8961=CARTESIAN_POINT('',(40.,0.24,-0.12));
#8962=CARTESIAN_POINT('Origin',(-0.1,0.42,0.3));
#8963=CARTESIAN_POINT('',(0.,0.42,0.3));
#8964=CARTESIAN_POINT('',(0.,0.42,0.15));
#8965=CARTESIAN_POINT('',(40.,0.42,0.3));
#8966=CARTESIAN_POINT('',(-0.1,0.42,0.3));
#8967=CARTESIAN_POINT('',(40.,0.42,0.15));
#8968=CARTESIAN_POINT('Origin',(-0.1,0.67,0.55));
#8969=CARTESIAN_POINT('',(0.,0.67,0.55));
#8970=CARTESIAN_POINT('',(6.93889390390723E-18,0.365,0.245));
#8971=CARTESIAN_POINT('',(40.,0.67,0.55));
#8972=CARTESIAN_POINT('',(-0.1,0.67,0.55));
#8973=CARTESIAN_POINT('',(40.,0.365,0.245));
#8974=CARTESIAN_POINT('Origin',(-0.1,0.82,0.55));
#8975=CARTESIAN_POINT('',(0.,0.82,0.55));
#8976=CARTESIAN_POINT('',(0.,0.41,0.55));
#8977=CARTESIAN_POINT('',(40.,0.82,0.55));
#8978=CARTESIAN_POINT('',(-0.1,0.82,0.55));
#8979=CARTESIAN_POINT('',(40.,0.41,0.55));
#8980=CARTESIAN_POINT('Origin',(-0.1,0.82,0.3));
#8981=CARTESIAN_POINT('',(0.,0.82,0.3));
#8982=CARTESIAN_POINT('',(0.,0.82,0.15));
#8983=CARTESIAN_POINT('',(40.,0.82,0.3));
#8984=CARTESIAN_POINT('',(-0.1,0.82,0.3));
#8985=CARTESIAN_POINT('',(40.,0.82,0.15));
#8986=CARTESIAN_POINT('Origin',(-0.1,1.05,0.3));
#8987=CARTESIAN_POINT('',(0.,1.,0.3));
#8988=CARTESIAN_POINT('',(0.,0.525,0.3));
#8989=CARTESIAN_POINT('',(40.,1.,0.3));
#8990=CARTESIAN_POINT('',(-0.05,1.,0.3));
#8991=CARTESIAN_POINT('',(40.,0.525,0.3));
#8992=CARTESIAN_POINT('Origin',(-0.1,-0.3,-0.82));
#8993=CARTESIAN_POINT('',(0.,-0.3,-0.82));
#8994=CARTESIAN_POINT('',(0.,-0.3,-1.));
#8995=CARTESIAN_POINT('',(0.,-0.3,-0.41));
#8996=CARTESIAN_POINT('',(40.,-0.3,-0.82));
#8997=CARTESIAN_POINT('',(-0.1,-0.3,-0.82));
#8998=CARTESIAN_POINT('',(40.,-0.3,-1.));
#8999=CARTESIAN_POINT('',(40.,-0.3,-0.41));
#9000=CARTESIAN_POINT('',(-0.05,-0.3,-1.));
#9001=CARTESIAN_POINT('Origin',(-0.1,-0.55,-0.82));
#9002=CARTESIAN_POINT('',(0.,-0.55,-0.82));
#9003=CARTESIAN_POINT('',(0.,-0.275,-0.82));
#9004=CARTESIAN_POINT('',(40.,-0.55,-0.82));
#9005=CARTESIAN_POINT('',(-0.1,-0.55,-0.82));
#9006=CARTESIAN_POINT('',(40.,-0.275,-0.82));
#9007=CARTESIAN_POINT('Origin',(-0.1,-0.55,-0.67));
#9008=CARTESIAN_POINT('',(0.,-0.55,-0.67));
#9009=CARTESIAN_POINT('',(0.,-0.55,-0.335));
#9010=CARTESIAN_POINT('',(40.,-0.55,-0.67));
#9011=CARTESIAN_POINT('',(-0.1,-0.55,-0.67));
#9012=CARTESIAN_POINT('',(40.,-0.55,-0.335));
#9013=CARTESIAN_POINT('Origin',(-0.1,-0.3,-0.42));
#9014=CARTESIAN_POINT('',(0.,-0.3,-0.42));
#9015=CARTESIAN_POINT('',(0.,-0.12,-0.24));
#9016=CARTESIAN_POINT('',(40.,-0.3,-0.42));
#9017=CARTESIAN_POINT('',(-0.1,-0.3,-0.42));
#9018=CARTESIAN_POINT('',(40.,-0.12,-0.24));
#9019=CARTESIAN_POINT('Origin',(-0.1,0.3,-0.42));
#9020=CARTESIAN_POINT('',(0.,0.3,-0.42));
#9021=CARTESIAN_POINT('',(0.,0.15,-0.42));
#9022=CARTESIAN_POINT('',(40.,0.3,-0.42));
#9023=CARTESIAN_POINT('',(-0.1,0.3,-0.42));
#9024=CARTESIAN_POINT('',(40.,0.15,-0.42));
#9025=CARTESIAN_POINT('Origin',(-0.1,0.55,-0.67));
#9026=CARTESIAN_POINT('',(0.,0.55,-0.67));
#9027=CARTESIAN_POINT('',(0.,0.245,-0.365));
#9028=CARTESIAN_POINT('',(40.,0.55,-0.67));
#9029=CARTESIAN_POINT('',(-0.1,0.55,-0.67));
#9030=CARTESIAN_POINT('',(40.,0.245,-0.365));
#9031=CARTESIAN_POINT('Origin',(-0.1,0.55,-0.82));
#9032=CARTESIAN_POINT('',(0.,0.55,-0.82));
#9033=CARTESIAN_POINT('',(0.,0.55,-0.41));
#9034=CARTESIAN_POINT('',(40.,0.55,-0.82));
#9035=CARTESIAN_POINT('',(-0.1,0.55,-0.82));
#9036=CARTESIAN_POINT('',(40.,0.55,-0.41));
#9037=CARTESIAN_POINT('Origin',(-0.1,0.3,-0.82));
#9038=CARTESIAN_POINT('',(0.,0.3,-0.82));
#9039=CARTESIAN_POINT('',(0.,0.15,-0.82));
#9040=CARTESIAN_POINT('',(40.,0.3,-0.82));
#9041=CARTESIAN_POINT('',(-0.1,0.3,-0.82));
#9042=CARTESIAN_POINT('',(40.,0.15,-0.82));
#9043=CARTESIAN_POINT('Origin',(-0.1,0.3,-1.05));
#9044=CARTESIAN_POINT('',(0.,0.3,-1.));
#9045=CARTESIAN_POINT('',(0.,0.3,-0.525));
#9046=CARTESIAN_POINT('',(40.,0.3,-1.));
#9047=CARTESIAN_POINT('',(-0.05,0.3,-1.));
#9048=CARTESIAN_POINT('',(40.,0.3,-0.525));
#9049=CARTESIAN_POINT('Origin',(-0.1,-0.82,0.3));
#9050=CARTESIAN_POINT('',(0.,-0.82,0.3));
#9051=CARTESIAN_POINT('',(0.,-1.,0.3));
#9052=CARTESIAN_POINT('',(0.,-0.41,0.3));
#9053=CARTESIAN_POINT('',(40.,-0.82,0.3));
#9054=CARTESIAN_POINT('',(-0.1,-0.82,0.3));
#9055=CARTESIAN_POINT('',(40.,-1.,0.3));
#9056=CARTESIAN_POINT('',(40.,-0.41,0.3));
#9057=CARTESIAN_POINT('',(-0.05,-1.,0.3));
#9058=CARTESIAN_POINT('Origin',(-0.1,-0.82,0.55));
#9059=CARTESIAN_POINT('',(0.,-0.82,0.55));
#9060=CARTESIAN_POINT('',(0.,-0.82,0.275));
#9061=CARTESIAN_POINT('',(40.,-0.82,0.55));
#9062=CARTESIAN_POINT('',(-0.1,-0.82,0.55));
#9063=CARTESIAN_POINT('',(40.,-0.82,0.275));
#9064=CARTESIAN_POINT('Origin',(-0.1,-0.67,0.55));
#9065=CARTESIAN_POINT('',(0.,-0.67,0.55));
#9066=CARTESIAN_POINT('',(0.,-0.335,0.55));
#9067=CARTESIAN_POINT('',(40.,-0.67,0.55));
#9068=CARTESIAN_POINT('',(-0.1,-0.67,0.55));
#9069=CARTESIAN_POINT('',(40.,-0.335,0.55));
#9070=CARTESIAN_POINT('Origin',(-0.1,-0.42,0.3));
#9071=CARTESIAN_POINT('',(0.,-0.42,0.3));
#9072=CARTESIAN_POINT('',(-6.93889390390723E-18,-0.24,0.12));
#9073=CARTESIAN_POINT('',(40.,-0.42,0.3));
#9074=CARTESIAN_POINT('',(-0.1,-0.42,0.3));
#9075=CARTESIAN_POINT('',(40.,-0.24,0.12));
#9076=CARTESIAN_POINT('Origin',(-0.1,-0.42,-0.3));
#9077=CARTESIAN_POINT('',(0.,-0.42,-0.3));
#9078=CARTESIAN_POINT('',(0.,-0.42,-0.15));
#9079=CARTESIAN_POINT('',(40.,-0.42,-0.3));
#9080=CARTESIAN_POINT('',(-0.1,-0.42,-0.3));
#9081=CARTESIAN_POINT('',(40.,-0.42,-0.15));
#9082=CARTESIAN_POINT('Origin',(-0.1,-0.67,-0.55));
#9083=CARTESIAN_POINT('',(0.,-0.67,-0.55));
#9084=CARTESIAN_POINT('',(0.,-0.365,-0.245));
#9085=CARTESIAN_POINT('',(40.,-0.67,-0.55));
#9086=CARTESIAN_POINT('',(-0.1,-0.67,-0.55));
#9087=CARTESIAN_POINT('',(40.,-0.365,-0.245));
#9088=CARTESIAN_POINT('Origin',(-0.1,-0.82,-0.55));
#9089=CARTESIAN_POINT('',(0.,-0.82,-0.55));
#9090=CARTESIAN_POINT('',(0.,-0.41,-0.55));
#9091=CARTESIAN_POINT('',(40.,-0.82,-0.55));
#9092=CARTESIAN_POINT('',(-0.1,-0.82,-0.55));
#9093=CARTESIAN_POINT('',(40.,-0.41,-0.55));
#9094=CARTESIAN_POINT('Origin',(-0.1,-0.82,-0.3));
#9095=CARTESIAN_POINT('',(0.,-0.82,-0.3));
#9096=CARTESIAN_POINT('',(0.,-0.82,-0.15));
#9097=CARTESIAN_POINT('',(40.,-0.82,-0.3));
#9098=CARTESIAN_POINT('',(-0.1,-0.82,-0.3));
#9099=CARTESIAN_POINT('',(40.,-0.82,-0.15));
#9100=CARTESIAN_POINT('Origin',(-0.1,-1.05,-0.3));
#9101=CARTESIAN_POINT('',(0.,-1.,-0.3));
#9102=CARTESIAN_POINT('',(0.,-0.525,-0.3));
#9103=CARTESIAN_POINT('',(40.,-1.,-0.3));
#9104=CARTESIAN_POINT('',(-0.05,-1.,-0.3));
#9105=CARTESIAN_POINT('',(40.,-0.525,-0.3));
#9106=CARTESIAN_POINT('Origin',(-0.1,0.3,0.82));
#9107=CARTESIAN_POINT('',(0.,0.3,0.82));
#9108=CARTESIAN_POINT('',(0.,0.3,1.));
#9109=CARTESIAN_POINT('',(0.,0.3,0.41));
#9110=CARTESIAN_POINT('',(40.,0.3,0.82));
#9111=CARTESIAN_POINT('',(-0.1,0.3,0.82));
#9112=CARTESIAN_POINT('',(40.,0.3,1.));
#9113=CARTESIAN_POINT('',(40.,0.3,0.41));
#9114=CARTESIAN_POINT('',(-0.05,0.3,1.));
#9115=CARTESIAN_POINT('Origin',(-0.1,0.55,0.82));
#9116=CARTESIAN_POINT('',(0.,0.55,0.82));
#9117=CARTESIAN_POINT('',(0.,0.275,0.82));
#9118=CARTESIAN_POINT('',(40.,0.55,0.82));
#9119=CARTESIAN_POINT('',(-0.1,0.55,0.82));
#9120=CARTESIAN_POINT('',(40.,0.275,0.82));
#9121=CARTESIAN_POINT('Origin',(-0.1,0.55,0.67));
#9122=CARTESIAN_POINT('',(0.,0.55,0.67));
#9123=CARTESIAN_POINT('',(0.,0.55,0.335));
#9124=CARTESIAN_POINT('',(40.,0.55,0.67));
#9125=CARTESIAN_POINT('',(-0.1,0.55,0.67));
#9126=CARTESIAN_POINT('',(40.,0.55,0.335));
#9127=CARTESIAN_POINT('Origin',(-0.1,0.3,0.42));
#9128=CARTESIAN_POINT('',(0.,0.3,0.42));
#9129=CARTESIAN_POINT('',(6.93889390390723E-18,0.12,0.24));
#9130=CARTESIAN_POINT('',(40.,0.3,0.42));
#9131=CARTESIAN_POINT('',(-0.1,0.3,0.42));
#9132=CARTESIAN_POINT('',(40.,0.12,0.24));
#9133=CARTESIAN_POINT('Origin',(-0.1,-0.3,0.42));
#9134=CARTESIAN_POINT('',(0.,-0.3,0.42));
#9135=CARTESIAN_POINT('',(0.,-0.15,0.42));
#9136=CARTESIAN_POINT('',(40.,-0.3,0.42));
#9137=CARTESIAN_POINT('',(-0.1,-0.3,0.42));
#9138=CARTESIAN_POINT('',(40.,-0.15,0.42));
#9139=CARTESIAN_POINT('Origin',(-0.1,-0.55,0.67));
#9140=CARTESIAN_POINT('',(0.,-0.55,0.67));
#9141=CARTESIAN_POINT('',(6.93889390390723E-18,-0.245,0.365));
#9142=CARTESIAN_POINT('',(40.,-0.55,0.67));
#9143=CARTESIAN_POINT('',(-0.1,-0.55,0.67));
#9144=CARTESIAN_POINT('',(40.,-0.245,0.365));
#9145=CARTESIAN_POINT('Origin',(-0.1,-0.55,0.82));
#9146=CARTESIAN_POINT('',(0.,-0.55,0.82));
#9147=CARTESIAN_POINT('',(0.,-0.55,0.41));
#9148=CARTESIAN_POINT('',(40.,-0.55,0.82));
#9149=CARTESIAN_POINT('',(-0.1,-0.55,0.82));
#9150=CARTESIAN_POINT('',(40.,-0.55,0.41));
#9151=CARTESIAN_POINT('Origin',(-0.1,-0.3,0.82));
#9152=CARTESIAN_POINT('',(0.,-0.3,0.82));
#9153=CARTESIAN_POINT('',(0.,-0.15,0.82));
#9154=CARTESIAN_POINT('',(40.,-0.3,0.82));
#9155=CARTESIAN_POINT('',(-0.1,-0.3,0.82));
#9156=CARTESIAN_POINT('',(40.,-0.15,0.82));
#9157=CARTESIAN_POINT('Origin',(-0.1,-0.3,1.05));
#9158=CARTESIAN_POINT('',(0.,-0.3,1.));
#9159=CARTESIAN_POINT('',(0.,-0.3,0.525));
#9160=CARTESIAN_POINT('',(40.,-0.3,1.));
#9161=CARTESIAN_POINT('',(-0.05,-0.3,1.));
#9162=CARTESIAN_POINT('',(40.,-0.3,0.525));
#9163=CARTESIAN_POINT('Origin',(-0.1,0.,0.));
#9164=CARTESIAN_POINT('',(40.,2.57175827820944E-17,0.21));
#9165=CARTESIAN_POINT('',(-0.1,-2.57175827820944E-17,0.21));
#9166=CARTESIAN_POINT('Origin',(40.,0.,0.));
#9167=CARTESIAN_POINT('Origin',(0.,1.,-1.));
#9168=CARTESIAN_POINT('',(0.,1.,1.));
#9169=CARTESIAN_POINT('',(0.,1.,-1.));
#9170=CARTESIAN_POINT('',(40.,1.,1.));
#9171=CARTESIAN_POINT('',(0.,1.,1.));
#9172=CARTESIAN_POINT('',(40.,1.,-1.));
#9173=CARTESIAN_POINT('Origin',(0.,1.,-1.));
#9174=CARTESIAN_POINT('',(40.,1.,-1.));
#9175=CARTESIAN_POINT('',(40.,1.,-1.));
#9176=CARTESIAN_POINT('',(0.,1.,-1.));
#9177=CARTESIAN_POINT('',(0.,1.,-1.));
#9178=CARTESIAN_POINT('',(0.,1.,-1.));
#9179=CARTESIAN_POINT('Origin',(0.,-1.,-1.));
#9180=CARTESIAN_POINT('',(0.,-1.,-1.));
#9181=CARTESIAN_POINT('',(40.,-1.,-1.));
#9182=CARTESIAN_POINT('Origin',(0.,-1.,-1.));
#9183=CARTESIAN_POINT('',(40.,-1.,-1.));
#9184=CARTESIAN_POINT('',(40.,-1.,-1.));
#9185=CARTESIAN_POINT('',(0.,-1.,-1.));
#9186=CARTESIAN_POINT('',(0.,-1.,-1.));
#9187=CARTESIAN_POINT('',(0.,-1.,-1.));
#9188=CARTESIAN_POINT('Origin',(0.,-1.,1.));
#9189=CARTESIAN_POINT('',(0.,-1.,1.));
#9190=CARTESIAN_POINT('',(40.,-1.,1.));
#9191=CARTESIAN_POINT('Origin',(0.,-1.,1.));
#9192=CARTESIAN_POINT('',(40.,-1.,1.));
#9193=CARTESIAN_POINT('',(40.,-1.,1.));
#9194=CARTESIAN_POINT('',(0.,-1.,1.));
#9195=CARTESIAN_POINT('',(0.,-1.,1.));
#9196=CARTESIAN_POINT('',(0.,-1.,1.));
#9197=CARTESIAN_POINT('Origin',(0.,1.,1.));
#9198=CARTESIAN_POINT('',(0.,1.,1.));
#9199=CARTESIAN_POINT('',(40.,1.,1.));
#9200=CARTESIAN_POINT('Origin',(0.,1.,1.));
#9201=CARTESIAN_POINT('',(40.,1.,1.));
#9202=CARTESIAN_POINT('',(0.,1.,1.));
#9203=CARTESIAN_POINT('Origin',(40.,0.,0.));
#9204=CARTESIAN_POINT('Origin',(0.,0.,0.));
#9986=UNCERTAINTY_MEASURE_WITH_UNIT(LENGTH_MEASURE(0.001),#10020,
'DISTANCE_ACCURACY_VALUE',
'Maximum model space distance between geometric entities at asserted c
onnectivities');
#9995=UNCERTAINTY_MEASURE_WITH_UNIT(LENGTH_MEASURE(0.001),#10020,
'DISTANCE_ACCURACY_VALUE',
'Maximum model space distance between geometric entities at asserted c
onnectivities');
#10010=(
GEOMETRIC_REPRESENTATION_CONTEXT(3)
GLOBAL_UNCERTAINTY_ASSIGNED_CONTEXT((#9986))
GLOBAL_UNIT_ASSIGNED_CONTEXT((#10020,#10022,#10023))
REPRESENTATION_CONTEXT('','3D')
);
#10019=(
GEOMETRIC_REPRESENTATION_CONTEXT(3)
GLOBAL_UNCERTAINTY_ASSIGNED_CONTEXT((#9995))
GLOBAL_UNIT_ASSIGNED_CONTEXT((#10020,#10022,#10023))
REPRESENTATION_CONTEXT('','3D')
);
#10020=(
LENGTH_UNIT()
NAMED_UNIT(*)
SI_UNIT(.CENTI.,.METRE.)
);
#10022=(
NAMED_UNIT(*)
PLANE_ANGLE_UNIT()
SI_UNIT($,.RADIAN.)
);
#10023=(
NAMED_UNIT(*)
SI_UNIT($,.STERADIAN.)
SOLID_ANGLE_UNIT()
);
#10038=SHAPE_DEFINITION_REPRESENTATION(#10061,#10181);
#10061=PRODUCT_DEFINITION_SHAPE('',$,#10205);
#10181=SHAPE_REPRESENTATION('',(#6066),#10010);
#10190=PRODUCT_DEFINITION_CONTEXT('part definition',#10261,'design');
#10205=PRODUCT_DEFINITION('Slotted Extrusion - 20 x 20 x 400 mm',
'Slotted Extrusion - 20 x 20 x 400 mm',#10228,#10190);
#10228=PRODUCT_DEFINITION_FORMATION('',$,#10277);
#10261=APPLICATION_CONTEXT(
'Core Data for Automotive Mechanical Design Process');
#10262=PRODUCT_CONTEXT('part definition',#10261,'mechanical');
#10277=PRODUCT('Slotted Extrusion - 20 x 20 x 400 mm',
'Slotted Extrusion - 20 x 20 x 400 mm',
'Slotted Extrusion - 20 x 20 x 400 mm',(#10262));
#10328=COLOUR_RGB('Light Blue',0.38,0.62,0.78);
#10329=FILL_AREA_STYLE_COLOUR('',#10328);
#10330=FILL_AREA_STYLE('',(#10329));
#10331=SURFACE_STYLE_FILL_AREA(#10330);
#10332=SURFACE_SIDE_STYLE('',(#10331));
#10333=SURFACE_STYLE_USAGE(.BOTH.,#10332);
#10334=PRESENTATION_STYLE_ASSIGNMENT((#10333));
ENDSEC;
END-ISO-10303-21;
